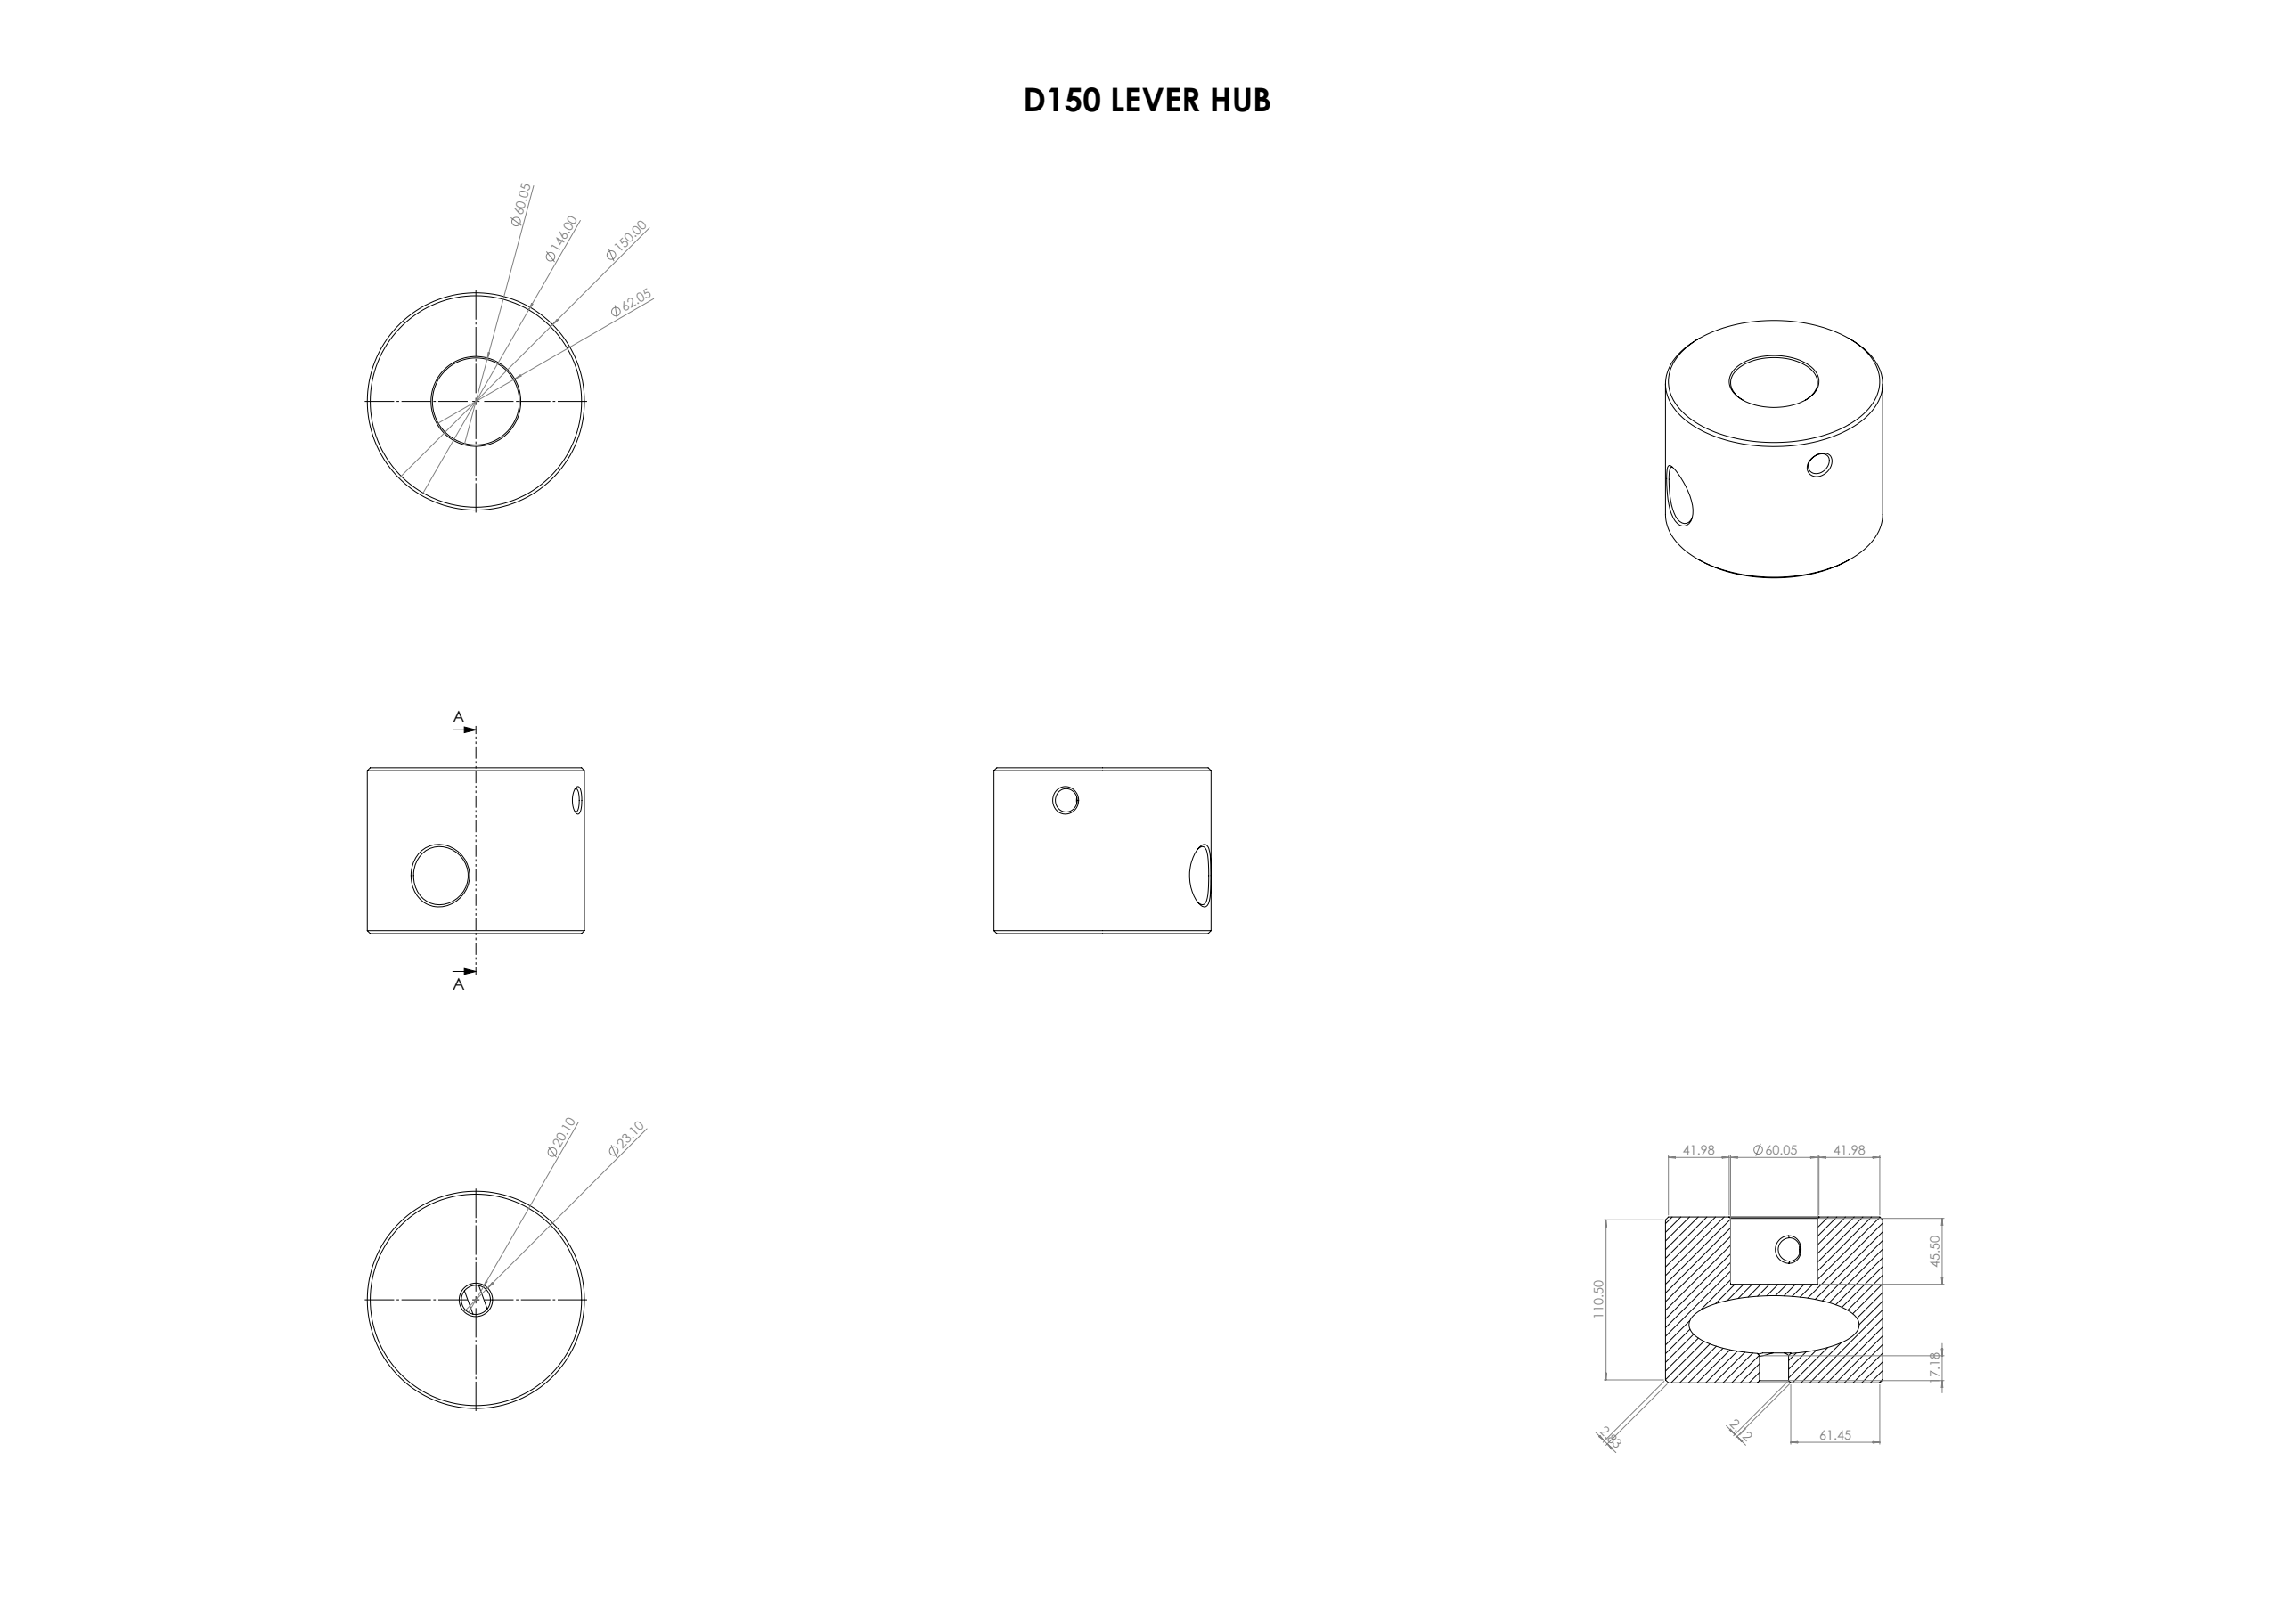
ISO-10303-21;
HEADER;
/* Generated by software containing ST-Developer
 * from STEP Tools, Inc. (www.steptools.com) 
 */

FILE_DESCRIPTION(
/* description */ (''),
/* implementation_level */ '2;1');

FILE_NAME(
/* name */ '04_D150_Lever_Hub.step',
/* time_stamp */ '2026-10-19T23:58:09-07:00',
/* author */ (''),
/* organization */ (''),
/* preprocessor_version */ 'ST-DEVELOPER v20.2',
/* originating_system */ 'Autodesk Translation Framework v15.15.0.0',
/* authorisation */ '');

FILE_SCHEMA (('AP203_CONFIGURATION_CONTROLLED_3D_DESIGN_OF_MECHANICAL_PARTS_AND_ASSEMBLIES_MIM_LF { 1 0 10303 203 3 1 4 }',
'AUTOMOTIVE_DESIGN { 1 0 10303 214 3 1 1 }','INTEGRATED_CNC_SCHEMA','MODEL_BASED_INTEGRATED_MANUFACTURING_SCHEMA',
'PROCESS_PLANNING_SCHEMA','AP242_MANAGED_MODEL_BASED_3D_ENGINEERING_MIM_LF { 1 0 10303 442 3 1 4 }'));
ENDSEC;

DATA;
#10=MECHANICAL_DESIGN_GEOMETRIC_PRESENTATION_REPRESENTATION('',(#417),#70757);
#280=B_SPLINE_SURFACE_WITH_KNOTS('',3,3,((#59484,#59485,#59486,#59487,#59488,
#59489,#59490,#59491,#59492,#59493,#59494,#59495,#59496,#59497,#59498,#59499,
#59500,#59501,#59502,#59503,#59504,#59505,#59506,#59507,#59508,#59509,#59510,
#59511,#59512,#59513,#59514,#59515,#59516,#59517,#59518,#59519,#59520,#59521,
#59522,#59523,#59524,#59525,#59526,#59527,#59528,#59529),(#59530,#59531,
#59532,#59533,#59534,#59535,#59536,#59537,#59538,#59539,#59540,#59541,#59542,
#59543,#59544,#59545,#59546,#59547,#59548,#59549,#59550,#59551,#59552,#59553,
#59554,#59555,#59556,#59557,#59558,#59559,#59560,#59561,#59562,#59563,#59564,
#59565,#59566,#59567,#59568,#59569,#59570,#59571,#59572,#59573,#59574,#59575),
(#59576,#59577,#59578,#59579,#59580,#59581,#59582,#59583,#59584,#59585,
#59586,#59587,#59588,#59589,#59590,#59591,#59592,#59593,#59594,#59595,#59596,
#59597,#59598,#59599,#59600,#59601,#59602,#59603,#59604,#59605,#59606,#59607,
#59608,#59609,#59610,#59611,#59612,#59613,#59614,#59615,#59616,#59617,#59618,
#59619,#59620,#59621),(#59622,#59623,#59624,#59625,#59626,#59627,#59628,
#59629,#59630,#59631,#59632,#59633,#59634,#59635,#59636,#59637,#59638,#59639,
#59640,#59641,#59642,#59643,#59644,#59645,#59646,#59647,#59648,#59649,#59650,
#59651,#59652,#59653,#59654,#59655,#59656,#59657,#59658,#59659,#59660,#59661,
#59662,#59663,#59664,#59665,#59666,#59667)),.UNSPECIFIED.,.F.,.T.,.F.,(4,
4),(4,1,1,1,1,1,1,1,1,1,1,1,1,1,1,1,1,1,1,1,1,1,1,1,1,1,1,1,1,1,1,1,1,1,
1,1,1,1,1,1,1,1,1,4),(0.,1.),(0.,0.434952646357303,0.869905292714605,1.08738161589326,
1.30485793907191,1.73981058542921,2.17476323178651,2.39223955496516,2.50097771655449,
2.55534679734915,2.60971587814382,3.04466852450112,3.15340668609044,3.47962117085842,
3.51586722472153,3.55211327858464,3.62460538631086,3.76958960176329,4.05955803266816,
4.34952646357303,4.6394948944779,4.92946332538276,5.21943175628763,5.5094001871925,
5.72687651037115,5.79936861809737,6.37930547990711,6.66927391081198,6.95924234171684,
7.24921077262171,7.53917920352658,7.82914763443145,8.11911606533632,8.26410028078875,
8.69905292714605,8.98902135805092,9.27898978895579,9.85892665076553,10.4388635125753,
10.8738161589326,10.9825543205219,11.3087688052899,11.7437214516472,12.1786740980045),
 .UNSPECIFIED.);
#281=B_SPLINE_SURFACE_WITH_KNOTS('',3,3,((#59965,#59966,#59967,#59968,#59969,
#59970,#59971,#59972,#59973,#59974,#59975,#59976,#59977,#59978,#59979,#59980,
#59981,#59982,#59983,#59984,#59985,#59986,#59987,#59988,#59989,#59990,#59991,
#59992,#59993,#59994,#59995,#59996,#59997,#59998,#59999,#60000,#60001,#60002,
#60003,#60004,#60005,#60006,#60007,#60008,#60009,#60010,#60011,#60012,#60013,
#60014,#60015,#60016,#60017,#60018),(#60019,#60020,#60021,#60022,#60023,
#60024,#60025,#60026,#60027,#60028,#60029,#60030,#60031,#60032,#60033,#60034,
#60035,#60036,#60037,#60038,#60039,#60040,#60041,#60042,#60043,#60044,#60045,
#60046,#60047,#60048,#60049,#60050,#60051,#60052,#60053,#60054,#60055,#60056,
#60057,#60058,#60059,#60060,#60061,#60062,#60063,#60064,#60065,#60066,#60067,
#60068,#60069,#60070,#60071,#60072),(#60073,#60074,#60075,#60076,#60077,
#60078,#60079,#60080,#60081,#60082,#60083,#60084,#60085,#60086,#60087,#60088,
#60089,#60090,#60091,#60092,#60093,#60094,#60095,#60096,#60097,#60098,#60099,
#60100,#60101,#60102,#60103,#60104,#60105,#60106,#60107,#60108,#60109,#60110,
#60111,#60112,#60113,#60114,#60115,#60116,#60117,#60118,#60119,#60120,#60121,
#60122,#60123,#60124,#60125,#60126),(#60127,#60128,#60129,#60130,#60131,
#60132,#60133,#60134,#60135,#60136,#60137,#60138,#60139,#60140,#60141,#60142,
#60143,#60144,#60145,#60146,#60147,#60148,#60149,#60150,#60151,#60152,#60153,
#60154,#60155,#60156,#60157,#60158,#60159,#60160,#60161,#60162,#60163,#60164,
#60165,#60166,#60167,#60168,#60169,#60170,#60171,#60172,#60173,#60174,#60175,
#60176,#60177,#60178,#60179,#60180)),.UNSPECIFIED.,.F.,.T.,.F.,(4,4),(4,
1,1,1,1,1,1,1,1,1,1,1,1,1,1,1,1,1,1,1,1,1,1,1,1,1,1,1,1,1,1,1,1,1,1,1,1,
1,1,1,1,1,1,1,1,1,1,1,1,1,1,4),(0.,1.),(0.,0.434952646357303,0.869905292714606,
1.08738161589326,1.30485793907191,1.73981058542921,1.84854874701854,2.17476323178651,
2.39223955496517,2.50097771655449,2.51456998675316,2.55534679734915,2.58253133774649,
2.60971587814382,2.88156128211713,3.04466852450112,3.47962117085842,3.51586722472153,
3.52492873818731,3.55211327858464,3.62460538631086,3.76958960176329,3.87832776335262,
4.05955803266816,4.34952646357303,4.6394948944779,4.85697121765655,4.92946332538276,
5.21943175628763,5.5094001871925,5.79936861809737,6.01684494127602,6.08933704900224,
6.37930547990711,6.95924234171684,7.03173444944306,7.24921077262171,7.53917920352658,
7.82914763443145,8.11911606533632,8.55406871169362,8.69905292714606,8.98902135805092,
9.27898978895579,9.64145032758688,9.85892665076553,10.4388635125753,10.8738161589326,
10.9825543205219,11.3087688052899,11.7437214516472,12.1786740980045),
 .UNSPECIFIED.);
#282=B_SPLINE_SURFACE_WITH_KNOTS('',3,3,((#60230,#60231,#60232,#60233,#60234,
#60235,#60236,#60237,#60238,#60239,#60240,#60241,#60242,#60243,#60244),
(#60245,#60246,#60247,#60248,#60249,#60250,#60251,#60252,#60253,#60254,
#60255,#60256,#60257,#60258,#60259),(#60260,#60261,#60262,#60263,#60264,
#60265,#60266,#60267,#60268,#60269,#60270,#60271,#60272,#60273,#60274),
(#60275,#60276,#60277,#60278,#60279,#60280,#60281,#60282,#60283,#60284,
#60285,#60286,#60287,#60288,#60289)),.UNSPECIFIED.,.F.,.F.,.F.,(4,4),(4,
1,1,1,1,1,1,1,2,2,4),(0.,1.),(0.442064469509103,0.769855887687593,1.09764730586608,
1.26154301495533,1.42543872404457,1.58933443313382,1.75323014222306,1.91712585131231,
2.08102156040155,2.14351932926336,2.6484237026181),.UNSPECIFIED.);
#283=B_SPLINE_SURFACE_WITH_KNOTS('',3,3,((#60302,#60303,#60304,#60305,#60306,
#60307,#60308,#60309,#60310,#60311,#60312,#60313,#60314,#60315),(#60316,
#60317,#60318,#60319,#60320,#60321,#60322,#60323,#60324,#60325,#60326,#60327,
#60328,#60329),(#60330,#60331,#60332,#60333,#60334,#60335,#60336,#60337,
#60338,#60339,#60340,#60341,#60342,#60343),(#60344,#60345,#60346,#60347,
#60348,#60349,#60350,#60351,#60352,#60353,#60354,#60355,#60356,#60357)),
 .UNSPECIFIED.,.F.,.F.,.F.,(4,4),(4,1,1,1,1,1,1,2,2,4),(0.,1.),(3.53272900796379,
3.8604875262342,4.18824604450462,4.35212530363983,4.51600456277503,4.72085363669404,
4.84376308104545,5.17152159931586,5.23401936817767,5.73877023945777),
 .UNSPECIFIED.);
#284=B_SPLINE_SURFACE_WITH_KNOTS('',3,3,((#60370,#60371,#60372,#60373,#60374,
#60375,#60376,#60377,#60378,#60379,#60380,#60381,#60382,#60383,#60384,#60385,
#60386,#60387,#60388,#60389,#60390,#60391,#60392,#60393),(#60394,#60395,
#60396,#60397,#60398,#60399,#60400,#60401,#60402,#60403,#60404,#60405,#60406,
#60407,#60408,#60409,#60410,#60411,#60412,#60413,#60414,#60415,#60416,#60417),
(#60418,#60419,#60420,#60421,#60422,#60423,#60424,#60425,#60426,#60427,
#60428,#60429,#60430,#60431,#60432,#60433,#60434,#60435,#60436,#60437,#60438,
#60439,#60440,#60441),(#60442,#60443,#60444,#60445,#60446,#60447,#60448,
#60449,#60450,#60451,#60452,#60453,#60454,#60455,#60456,#60457,#60458,#60459,
#60460,#60461,#60462,#60463,#60464,#60465)),.UNSPECIFIED.,.F.,.T.,.F.,(4,
4),(4,1,1,1,1,2,2,1,2,1,1,1,1,1,1,1,1,1,4),(0.,1.),(-3.74583112016425,-3.27642035446956,
-3.15906766304589,-2.80700958877487,-2.33759882308018,-1.86818805738549,
-1.79629199573878,-1.50783982646145,-1.21938765718412,-0.911365009587737,
-0.757353685789545,-0.603342361991352,-0.295319714394966,-0.141308390596773,
0.0127029332014201,0.320725580797806,0.628748228394192,0.936770875990578,
1.24479352358696),.UNSPECIFIED.);
#285=B_SPLINE_SURFACE_WITH_KNOTS('',3,3,((#60599,#60600,#60601,#60602,#60603,
#60604,#60605,#60606,#60607,#60608,#60609,#60610,#60611,#60612,#60613,#60614,
#60615,#60616,#60617,#60618,#60619,#60620,#60621,#60622,#60623,#60624,#60625,
#60626,#60627,#60628,#60629,#60630,#60631,#60632,#60633,#60634,#60635,#60636,
#60637,#60638,#60639,#60640,#60641,#60642,#60643,#60644,#60645,#60646,#60647,
#60648,#60649,#60650,#60651,#60652,#60653,#60654,#60655,#60656),(#60657,
#60658,#60659,#60660,#60661,#60662,#60663,#60664,#60665,#60666,#60667,#60668,
#60669,#60670,#60671,#60672,#60673,#60674,#60675,#60676,#60677,#60678,#60679,
#60680,#60681,#60682,#60683,#60684,#60685,#60686,#60687,#60688,#60689,#60690,
#60691,#60692,#60693,#60694,#60695,#60696,#60697,#60698,#60699,#60700,#60701,
#60702,#60703,#60704,#60705,#60706,#60707,#60708,#60709,#60710,#60711,#60712,
#60713,#60714),(#60715,#60716,#60717,#60718,#60719,#60720,#60721,#60722,
#60723,#60724,#60725,#60726,#60727,#60728,#60729,#60730,#60731,#60732,#60733,
#60734,#60735,#60736,#60737,#60738,#60739,#60740,#60741,#60742,#60743,#60744,
#60745,#60746,#60747,#60748,#60749,#60750,#60751,#60752,#60753,#60754,#60755,
#60756,#60757,#60758,#60759,#60760,#60761,#60762,#60763,#60764,#60765,#60766,
#60767,#60768,#60769,#60770,#60771,#60772),(#60773,#60774,#60775,#60776,
#60777,#60778,#60779,#60780,#60781,#60782,#60783,#60784,#60785,#60786,#60787,
#60788,#60789,#60790,#60791,#60792,#60793,#60794,#60795,#60796,#60797,#60798,
#60799,#60800,#60801,#60802,#60803,#60804,#60805,#60806,#60807,#60808,#60809,
#60810,#60811,#60812,#60813,#60814,#60815,#60816,#60817,#60818,#60819,#60820,
#60821,#60822,#60823,#60824,#60825,#60826,#60827,#60828,#60829,#60830)),
 .UNSPECIFIED.,.F.,.T.,.F.,(4,4),(4,1,1,1,1,1,1,1,1,1,1,1,1,1,1,1,1,1,1,
1,1,1,1,1,1,1,1,1,1,1,1,1,1,1,1,1,1,1,1,1,1,1,1,1,1,1,1,1,1,1,1,1,1,1,1,
4),(0.,1.),(0.,0.173419326361772,0.346838652723544,0.520257979085315,0.693677305447087,
0.867096631808859,0.953806294989745,0.997161126580188,1.04051595817063,
1.38735461089417,1.41625783195447,1.44516105301476,1.50296749513536,1.61858037937654,
1.73419326361772,1.8498061478589,2.08103191634126,2.10993513740156,2.13883835846185,
2.19664480058244,2.25445124270303,2.28335446376333,2.31225768482362,2.54348345330599,
2.57238667436628,2.60128989542658,2.65909633754717,2.77470922178835,2.94812854815012,
3.12154787451189,3.20825753769278,3.29496720087366,3.38167686405455,3.39251557195216,
3.40335427984977,3.42503169564499,3.4358704035426,3.44670911144021,3.45754781933783,
3.46296717328663,3.46838652723544,3.64180585359721,3.81522517995898,3.82606388785659,
3.8369025957542,3.85858001154942,3.90193484313987,3.98864450632075,4.07535416950164,
4.16206383268252,4.33548315904429,4.35716057483952,4.37883799063474,4.42219282222518,
4.50890248540607,4.85574113812961),.UNSPECIFIED.);
#387=SHAPE_REPRESENTATION_RELATIONSHIP('SRR','None',#70828,#402);
#402=ADVANCED_BREP_SHAPE_REPRESENTATION('',(#477),#70752);
#417=STYLED_ITEM('',(#71033),#477);
#477=MANIFOLD_SOLID_BREP('Hub',#26882);
#723=CYLINDRICAL_SURFACE('',#27792,7.5);
#724=CYLINDRICAL_SURFACE('',#27795,2.01);
#725=CYLINDRICAL_SURFACE('',#27799,1.005);
#726=CYLINDRICAL_SURFACE('',#27805,0.805000000000009);
#727=CYLINDRICAL_SURFACE('',#27806,3.0025);
#868=FACE_BOUND('',#4617,.T.);
#869=FACE_BOUND('',#4618,.T.);
#870=FACE_BOUND('',#4619,.T.);
#871=FACE_BOUND('',#4621,.T.);
#872=FACE_BOUND('',#4626,.T.);
#873=FACE_BOUND('',#4632,.T.);
#874=FACE_BOUND('',#4639,.T.);
#1376=B_SPLINE_CURVE_WITH_KNOTS('',3,(#59671,#59672,#59673,#59674,#59675,
#59676,#59677,#59678,#59679,#59680,#59681,#59682,#59683,#59684,#59685,#59686,
#59687,#59688,#59689,#59690,#59691,#59692,#59693,#59694,#59695,#59696,#59697,
#59698,#59699,#59700,#59701,#59702,#59703,#59704,#59705,#59706,#59707,#59708,
#59709,#59710,#59711,#59712,#59713,#59714,#59715,#59716),.UNSPECIFIED.,
 .T.,.F.,(4,1,1,1,1,1,1,1,1,1,1,1,1,1,1,1,1,1,1,1,1,1,1,1,1,1,1,1,1,1,1,
1,1,1,1,1,1,1,1,1,1,1,1,4),(0.,0.434952646357303,0.869905292714605,1.08738161589326,
1.30485793907191,1.73981058542921,2.17476323178651,2.39223955496516,2.50097771655449,
2.55534679734915,2.60971587814382,3.04466852450112,3.15340668609044,3.47962117085842,
3.51586722472153,3.55211327858464,3.62460538631086,3.76958960176329,4.05955803266816,
4.34952646357303,4.6394948944779,4.92946332538276,5.21943175628763,5.5094001871925,
5.72687651037115,5.79936861809737,6.37930547990711,6.66927391081198,6.95924234171684,
7.24921077262171,7.53917920352658,7.82914763443145,8.11911606533632,8.26410028078875,
8.69905292714605,8.98902135805092,9.27898978895579,9.85892665076553,10.4388635125753,
10.8738161589326,10.9825543205219,11.3087688052899,11.7437214516472,12.1786740980045),
 .UNSPECIFIED.);
#1377=B_SPLINE_CURVE_WITH_KNOTS('',3,(#59717,#59718,#59719,#59720,#59721,
#59722,#59723,#59724,#59725,#59726,#59727,#59728,#59729,#59730,#59731,#59732,
#59733,#59734,#59735,#59736,#59737,#59738,#59739,#59740,#59741,#59742,#59743,
#59744,#59745,#59746,#59747,#59748,#59749,#59750,#59751,#59752,#59753,#59754,
#59755,#59756,#59757,#59758,#59759,#59760,#59761,#59762),.UNSPECIFIED.,
 .T.,.F.,(4,1,1,1,1,1,1,1,1,1,1,1,1,1,1,1,1,1,1,1,1,1,1,1,1,1,1,1,1,1,1,
1,1,1,1,1,1,1,1,1,1,1,1,4),(-12.1786740980045,-11.7437214516472,-11.3087688052899,
-10.9825543205219,-10.8738161589326,-10.4388635125753,-9.85892665076553,
-9.27898978895579,-8.98902135805092,-8.69905292714605,-8.26410028078875,
-8.11911606533632,-7.82914763443145,-7.53917920352658,-7.24921077262171,
-6.95924234171684,-6.66927391081198,-6.37930547990711,-5.79936861809737,
-5.72687651037115,-5.5094001871925,-5.21943175628763,-4.92946332538276,
-4.6394948944779,-4.34952646357303,-4.05955803266816,-3.76958960176329,
-3.62460538631086,-3.55211327858464,-3.51586722472153,-3.47962117085842,
-3.15340668609044,-3.04466852450112,-2.60971587814382,-2.55534679734915,
-2.50097771655449,-2.39223955496516,-2.17476323178651,-1.73981058542921,
-1.30485793907191,-1.08738161589326,-0.869905292714605,-0.434952646357303,
0.),.UNSPECIFIED.);
#1378=B_SPLINE_CURVE_WITH_KNOTS('',3,(#59770,#59771,#59772,#59773,#59774,
#59775,#59776,#59777,#59778,#59779,#59780,#59781,#59782,#59783,#59784,#59785,
#59786,#59787,#59788,#59789,#59790,#59791,#59792,#59793,#59794,#59795,#59796,
#59797,#59798,#59799,#59800,#59801,#59802,#59803,#59804,#59805,#59806,#59807,
#59808,#59809,#59810,#59811,#59812,#59813,#59814,#59815,#59816,#59817,#59818,
#59819,#59820,#59821,#59822,#59823),.UNSPECIFIED.,.T.,.F.,(4,1,1,1,1,1,
1,1,1,1,1,1,1,1,1,1,1,1,1,1,1,1,1,1,1,1,1,1,1,1,1,1,1,1,1,1,1,1,1,1,1,1,
1,1,1,1,1,1,1,1,1,4),(-12.1786740980045,-11.7437214516472,-11.3087688052899,
-10.9825543205219,-10.8738161589326,-10.4388635125753,-9.85892665076553,
-9.64145032758688,-9.27898978895579,-8.98902135805092,-8.69905292714606,
-8.55406871169362,-8.11911606533632,-7.82914763443145,-7.53917920352658,
-7.24921077262171,-7.03173444944306,-6.95924234171684,-6.37930547990711,
-6.08933704900224,-6.01684494127602,-5.79936861809737,-5.5094001871925,
-5.21943175628763,-4.92946332538276,-4.85697121765655,-4.6394948944779,
-4.34952646357303,-4.05955803266816,-3.87832776335262,-3.76958960176329,
-3.62460538631086,-3.55211327858464,-3.52492873818731,-3.51586722472153,
-3.47962117085842,-3.04466852450112,-2.88156128211713,-2.60971587814382,
-2.58253133774649,-2.55534679734915,-2.51456998675316,-2.50097771655449,
-2.39223955496517,-2.17476323178651,-1.84854874701854,-1.73981058542921,
-1.30485793907191,-1.08738161589326,-0.869905292714606,-0.434952646357303,
0.),.UNSPECIFIED.);
#1379=B_SPLINE_CURVE_WITH_KNOTS('',3,(#59825,#59826,#59827,#59828,#59829,
#59830,#59831,#59832,#59833,#59834,#59835,#59836,#59837,#59838,#59839,#59840,
#59841,#59842,#59843,#59844,#59845,#59846,#59847,#59848,#59849,#59850,#59851,
#59852,#59853,#59854,#59855,#59856,#59857,#59858,#59859,#59860,#59861,#59862,
#59863,#59864,#59865,#59866,#59867,#59868,#59869,#59870,#59871,#59872,#59873,
#59874,#59875,#59876,#59877,#59878,#59879,#59880,#59881,#59882),
 .UNSPECIFIED.,.T.,.F.,(4,1,1,1,1,1,1,1,1,1,1,1,1,1,1,1,1,1,1,1,1,1,1,1,
1,1,1,1,1,1,1,1,1,1,1,1,1,1,1,1,1,1,1,1,1,1,1,1,1,1,1,1,1,1,1,4),(-4.85574113812961,
-4.50890248540607,-4.42219282222518,-4.37883799063474,-4.35716057483952,
-4.33548315904429,-4.16206383268252,-4.07535416950164,-3.98864450632075,
-3.90193484313987,-3.85858001154942,-3.8369025957542,-3.82606388785659,
-3.81522517995898,-3.64180585359721,-3.46838652723544,-3.46296717328663,
-3.45754781933783,-3.44670911144021,-3.4358704035426,-3.42503169564499,
-3.40335427984977,-3.39251557195216,-3.38167686405455,-3.29496720087366,
-3.20825753769278,-3.12154787451189,-2.94812854815012,-2.77470922178835,
-2.65909633754717,-2.60128989542658,-2.57238667436628,-2.54348345330599,
-2.31225768482362,-2.28335446376333,-2.25445124270303,-2.19664480058244,
-2.13883835846185,-2.10993513740156,-2.08103191634126,-1.8498061478589,
-1.73419326361772,-1.61858037937654,-1.50296749513536,-1.44516105301476,
-1.41625783195447,-1.38735461089417,-1.04051595817063,-0.997161126580188,
-0.953806294989745,-0.867096631808859,-0.693677305447087,-0.520257979085315,
-0.346838652723544,-0.173419326361772,0.),.UNSPECIFIED.);
#1380=B_SPLINE_CURVE_WITH_KNOTS('',3,(#59886,#59887,#59888,#59889,#59890,
#59891,#59892,#59893,#59894,#59895,#59896,#59897,#59898,#59899,#59900,#59901,
#59902,#59903,#59904,#59905,#59906,#59907,#59908,#59909,#59910,#59911,#59912,
#59913,#59914,#59915,#59916,#59917,#59918,#59919,#59920,#59921,#59922,#59923,
#59924,#59925,#59926,#59927,#59928,#59929,#59930,#59931,#59932,#59933,#59934,
#59935,#59936,#59937,#59938,#59939),.UNSPECIFIED.,.T.,.F.,(4,1,1,1,1,1,
1,1,1,1,1,1,1,1,1,1,1,1,1,1,1,1,1,1,1,1,1,1,1,1,1,1,1,1,1,1,1,1,1,1,1,1,
1,1,1,1,1,1,1,1,1,4),(0.,0.434952646357303,0.869905292714606,1.08738161589326,
1.30485793907191,1.73981058542921,1.84854874701854,2.17476323178651,2.39223955496517,
2.50097771655449,2.51456998675316,2.55534679734915,2.58253133774649,2.60971587814382,
2.88156128211713,3.04466852450112,3.47962117085842,3.51586722472153,3.52492873818731,
3.55211327858464,3.62460538631086,3.76958960176329,3.87832776335262,4.05955803266816,
4.34952646357303,4.6394948944779,4.85697121765655,4.92946332538276,5.21943175628763,
5.5094001871925,5.79936861809737,6.01684494127602,6.08933704900224,6.37930547990711,
6.95924234171684,7.03173444944306,7.24921077262171,7.53917920352658,7.82914763443145,
8.11911606533632,8.55406871169362,8.69905292714606,8.98902135805092,9.27898978895579,
9.64145032758688,9.85892665076553,10.4388635125753,10.8738161589326,10.9825543205219,
11.3087688052899,11.7437214516472,12.1786740980045),.UNSPECIFIED.);
#1381=B_SPLINE_CURVE_WITH_KNOTS('',3,(#59944,#59945,#59946,#59947,#59948,
#59949,#59950,#59951,#59952),.UNSPECIFIED.,.F.,.F.,(4,1,1,1,1,1,4),(-5.09886318526994,
-4.84376308104545,-4.72085363669404,-4.51600456277503,-4.35212530363983,
-4.18824604450462,-4.17262768684822),.UNSPECIFIED.);
#1382=B_SPLINE_CURVE_WITH_KNOTS('',3,(#59955,#59956,#59957,#59958,#59959,
#59960,#59961,#59962,#59963,#59964),.UNSPECIFIED.,.F.,.F.,(4,1,1,1,1,1,
1,4),(-2.00844283647624,-1.91712585131231,-1.75323014222306,-1.58933443313382,
-1.42543872404457,-1.26154301495533,-1.09764730586608,-1.08195609140638),
 .UNSPECIFIED.);
#1383=B_SPLINE_CURVE_WITH_KNOTS('',3,(#60191,#60192,#60193,#60194,#60195,
#60196,#60197,#60198,#60199,#60200,#60201,#60202,#60203,#60204,#60205),
 .UNSPECIFIED.,.F.,.F.,(4,1,1,1,1,1,1,1,2,2,4),(0.442064469509103,0.769855887687593,
1.09764730586608,1.26154301495533,1.42543872404457,1.58933443313382,1.75323014222306,
1.91712585131231,2.08102156040155,2.14351932926336,2.6484237026181),
 .UNSPECIFIED.);
#1384=B_SPLINE_CURVE_WITH_KNOTS('',3,(#60209,#60210,#60211,#60212,#60213,
#60214,#60215,#60216,#60217,#60218,#60219,#60220,#60221,#60222),
 .UNSPECIFIED.,.F.,.F.,(4,1,1,1,1,1,1,2,2,4),(3.53272900796379,3.8604875262342,
4.18824604450462,4.35212530363983,4.51600456277503,4.72085363669404,4.84376308104545,
5.17152159931586,5.23401936817767,5.73877023945777),.UNSPECIFIED.);
#1385=B_SPLINE_CURVE_WITH_KNOTS('',3,(#60290,#60291,#60292,#60293,#60294,
#60295),.UNSPECIFIED.,.F.,.F.,(4,2,4),(0.,0.395295738561713,0.750556975338415),
 .UNSPECIFIED.);
#1386=B_SPLINE_CURVE_WITH_KNOTS('',3,(#60296,#60297,#60298,#60299,#60300,
#60301),.UNSPECIFIED.,.F.,.F.,(4,2,4),(0.,0.242165599626981,0.747632926534989),
 .UNSPECIFIED.);
#1387=B_SPLINE_CURVE_WITH_KNOTS('',3,(#60358,#60359,#60360,#60361,#60362,
#60363),.UNSPECIFIED.,.F.,.F.,(4,2,4),(0.,0.395285417853985,0.750556986687262),
 .UNSPECIFIED.);
#1388=B_SPLINE_CURVE_WITH_KNOTS('',3,(#60364,#60365,#60366,#60367,#60368,
#60369),.UNSPECIFIED.,.F.,.F.,(4,2,4),(0.,0.242119658779455,0.747632520146835),
 .UNSPECIFIED.);
#1389=B_SPLINE_CURVE_WITH_KNOTS('',3,(#60470,#60471,#60472,#60473,#60474,
#60475,#60476,#60477,#60478,#60479,#60480,#60481,#60482,#60483,#60484,#60485,
#60486,#60487,#60488,#60489,#60490),.UNSPECIFIED.,.F.,.F.,(4,1,1,1,1,2,
2,1,2,1,1,1,1,1,1,4),(-3.74583112016425,-3.27642035446956,-3.15906766304589,
-2.80700958877487,-2.33759882308018,-1.86818805738549,-1.79629199573878,
-1.50783982646145,-1.21938765718412,-0.911365009587737,-0.757353685789545,
-0.603342361991352,-0.295319714394966,-0.141308390596773,0.0127029332014201,
0.0186613584180625),.UNSPECIFIED.);
#1390=B_SPLINE_CURVE_WITH_KNOTS('',3,(#60491,#60492,#60493,#60494,#60495,
#60496,#60497),.UNSPECIFIED.,.F.,.F.,(4,1,1,1,4),(0.0186613584180625,0.320725580797806,
0.628748228394192,0.936770875990578,1.24479352358696),.UNSPECIFIED.);
#1391=B_SPLINE_CURVE_WITH_KNOTS('',3,(#60499,#60500,#60501,#60502,#60503,
#60504,#60505,#60506,#60507,#60508,#60509),.UNSPECIFIED.,.F.,.F.,(4,1,1,
1,1,1,1,1,4),(-1.24479352358696,-0.936770875990578,-0.628748228394192,-0.320725580797806,
-0.0127029332014201,0.141308390596773,0.295319714394966,0.603342361991352,
0.74818116877789),.UNSPECIFIED.);
#1392=B_SPLINE_CURVE_WITH_KNOTS('',3,(#60511,#60512,#60513,#60514,#60515,
#60516,#60517,#60518,#60519),.UNSPECIFIED.,.F.,.F.,(4,1,1,2,1,4),(0.74818116877789,
0.757353685789545,0.911365009587737,1.21938765718412,1.50783982646145,1.69059414559038),
 .UNSPECIFIED.);
#1393=B_SPLINE_CURVE_WITH_KNOTS('',3,(#60520,#60521,#60522,#60523,#60524,
#60525,#60526,#60527,#60528,#60529,#60530,#60531),.UNSPECIFIED.,.F.,.F.,
(4,2,2,1,1,1,1,4),(1.69059414559038,1.79629199573878,1.86818805738549,2.33759882308018,
2.80700958877487,3.15906766304589,3.27642035446956,3.74583112016425),
 .UNSPECIFIED.);
#1394=B_SPLINE_CURVE_WITH_KNOTS('',3,(#60534,#60535,#60536,#60537,#60538,
#60539,#60540,#60541,#60542,#60543,#60544,#60545,#60546,#60547,#60548,#60549,
#60550,#60551,#60552,#60553,#60554,#60555,#60556,#60557,#60558,#60559,#60560,
#60561,#60562,#60563,#60564,#60565,#60566,#60567,#60568,#60569,#60570,#60571,
#60572,#60573,#60574,#60575,#60576,#60577,#60578,#60579,#60580,#60581,#60582,
#60583,#60584,#60585,#60586,#60587,#60588,#60589,#60590,#60591),
 .UNSPECIFIED.,.T.,.F.,(4,1,1,1,1,1,1,1,1,1,1,1,1,1,1,1,1,1,1,1,1,1,1,1,
1,1,1,1,1,1,1,1,1,1,1,1,1,1,1,1,1,1,1,1,1,1,1,1,1,1,1,1,1,1,1,4),(0.,0.173419326361772,
0.346838652723544,0.520257979085315,0.693677305447087,0.867096631808859,
0.953806294989745,0.997161126580188,1.04051595817063,1.38735461089417,1.41625783195447,
1.44516105301476,1.50296749513536,1.61858037937654,1.73419326361772,1.8498061478589,
2.08103191634126,2.10993513740156,2.13883835846185,2.19664480058244,2.25445124270303,
2.28335446376333,2.31225768482362,2.54348345330599,2.57238667436628,2.60128989542658,
2.65909633754717,2.77470922178835,2.94812854815012,3.12154787451189,3.20825753769278,
3.29496720087366,3.38167686405455,3.39251557195216,3.40335427984977,3.42503169564499,
3.4358704035426,3.44670911144021,3.45754781933783,3.46296717328663,3.46838652723544,
3.64180585359721,3.81522517995898,3.82606388785659,3.8369025957542,3.85858001154942,
3.90193484313987,3.98864450632075,4.07535416950164,4.16206383268252,4.33548315904429,
4.35716057483952,4.37883799063474,4.42219282222518,4.50890248540607,4.85574113812961),
 .UNSPECIFIED.);
#1911=PLANE('',#27803);
#1912=PLANE('',#27809);
#1913=PLANE('',#27810);
#1914=PLANE('',#27811);
#1915=PLANE('',#27814);
#3103=FACE_OUTER_BOUND('',#4615,.T.);
#3104=FACE_OUTER_BOUND('',#4616,.T.);
#3105=FACE_OUTER_BOUND('',#4620,.T.);
#3106=FACE_OUTER_BOUND('',#4622,.T.);
#3107=FACE_OUTER_BOUND('',#4623,.T.);
#3108=FACE_OUTER_BOUND('',#4624,.T.);
#3109=FACE_OUTER_BOUND('',#4625,.T.);
#3110=FACE_OUTER_BOUND('',#4627,.T.);
#3111=FACE_OUTER_BOUND('',#4628,.T.);
#3112=FACE_OUTER_BOUND('',#4629,.T.);
#3113=FACE_OUTER_BOUND('',#4630,.T.);
#3114=FACE_OUTER_BOUND('',#4631,.T.);
#3115=FACE_OUTER_BOUND('',#4633,.T.);
#3116=FACE_OUTER_BOUND('',#4634,.T.);
#3117=FACE_OUTER_BOUND('',#4635,.T.);
#3118=FACE_OUTER_BOUND('',#4636,.T.);
#3119=FACE_OUTER_BOUND('',#4637,.T.);
#3120=FACE_OUTER_BOUND('',#4638,.T.);
#3121=FACE_OUTER_BOUND('',#4640,.T.);
#3122=FACE_OUTER_BOUND('',#4641,.T.);
#4615=EDGE_LOOP('',(#20248,#20249,#20250,#20251));
#4616=EDGE_LOOP('',(#20252,#20253,#20254,#20255));
#4617=EDGE_LOOP('',(#20256));
#4618=EDGE_LOOP('',(#20257));
#4619=EDGE_LOOP('',(#20258));
#4620=EDGE_LOOP('',(#20259,#20260,#20261,#20262));
#4621=EDGE_LOOP('',(#20263,#20264,#20265,#20266));
#4622=EDGE_LOOP('',(#20267,#20268,#20269,#20270));
#4623=EDGE_LOOP('',(#20271,#20272,#20273,#20274));
#4624=EDGE_LOOP('',(#20275,#20276,#20277,#20278,#20279,#20280,#20281,#20282));
#4625=EDGE_LOOP('',(#20283));
#4626=EDGE_LOOP('',(#20284));
#4627=EDGE_LOOP('',(#20285,#20286,#20287,#20288));
#4628=EDGE_LOOP('',(#20289,#20290,#20291,#20292));
#4629=EDGE_LOOP('',(#20293,#20294,#20295,#20296,#20297,#20298,#20299));
#4630=EDGE_LOOP('',(#20300,#20301,#20302,#20303,#20304));
#4631=EDGE_LOOP('',(#20305,#20306,#20307,#20308));
#4632=EDGE_LOOP('',(#20309,#20310,#20311));
#4633=EDGE_LOOP('',(#20312,#20313,#20314,#20315));
#4634=EDGE_LOOP('',(#20316,#20317,#20318,#20319,#20320));
#4635=EDGE_LOOP('',(#20321,#20322,#20323,#20324));
#4636=EDGE_LOOP('',(#20325));
#4637=EDGE_LOOP('',(#20326,#20327,#20328,#20329));
#4638=EDGE_LOOP('',(#20330));
#4639=EDGE_LOOP('',(#20331));
#4640=EDGE_LOOP('',(#20332,#20333,#20334,#20335));
#4641=EDGE_LOOP('',(#20336,#20337,#20338,#20339));
#6234=LINE('',#59670,#8731);
#6235=LINE('',#59767,#8732);
#6236=LINE('',#59885,#8733);
#6237=LINE('',#59942,#8734);
#6238=LINE('',#59954,#8735);
#6239=LINE('',#60181,#8736);
#6240=LINE('',#60186,#8737);
#6241=LINE('',#60225,#8738);
#6242=LINE('',#60468,#8739);
#6243=LINE('',#60592,#8740);
#6244=LINE('',#60597,#8741);
#6245=LINE('',#60831,#8742);
#6246=LINE('',#60837,#8743);
#6247=LINE('',#60843,#8744);
#6248=LINE('',#60845,#8745);
#8731=VECTOR('',#31067,1.);
#8732=VECTOR('',#31072,7.5);
#8733=VECTOR('',#31077,2.01);
#8734=VECTOR('',#31078,1.);
#8735=VECTOR('',#31079,1.);
#8736=VECTOR('',#31080,1.);
#8737=VECTOR('',#31085,1.08);
#8738=VECTOR('',#31094,1.005);
#8739=VECTOR('',#31101,1.);
#8740=VECTOR('',#31104,0.805000000000009);
#8741=VECTOR('',#31109,3.0025);
#8742=VECTOR('',#31112,1.);
#8743=VECTOR('',#31121,3.0525);
#8744=VECTOR('',#31130,7.4);
#8745=VECTOR('',#31133,7.4);
#10864=CIRCLE('',#27793,7.5);
#10865=CIRCLE('',#27794,7.5);
#10866=CIRCLE('',#27797,1.155);
#10867=CIRCLE('',#27798,1.005);
#10868=CIRCLE('',#27800,1.005);
#10869=CIRCLE('',#27801,1.005);
#10870=CIRCLE('',#27802,1.005);
#10871=CIRCLE('',#27804,7.3);
#10872=CIRCLE('',#27807,3.0025);
#10873=CIRCLE('',#27808,3.0025);
#10874=CIRCLE('',#27813,3.1025);
#10875=CIRCLE('',#27815,7.3);
#12004=VERTEX_POINT('',#59668);
#12005=VERTEX_POINT('',#59669);
#12006=VERTEX_POINT('',#59764);
#12007=VERTEX_POINT('',#59766);
#12008=VERTEX_POINT('',#59769);
#12009=VERTEX_POINT('',#59824);
#12010=VERTEX_POINT('',#59884);
#12011=VERTEX_POINT('',#59940);
#12012=VERTEX_POINT('',#59941);
#12013=VERTEX_POINT('',#59943);
#12014=VERTEX_POINT('',#59953);
#12015=VERTEX_POINT('',#60183);
#12016=VERTEX_POINT('',#60185);
#12017=VERTEX_POINT('',#60189);
#12018=VERTEX_POINT('',#60190);
#12019=VERTEX_POINT('',#60206);
#12020=VERTEX_POINT('',#60208);
#12021=VERTEX_POINT('',#60223);
#12022=VERTEX_POINT('',#60228);
#12023=VERTEX_POINT('',#60466);
#12024=VERTEX_POINT('',#60467);
#12025=VERTEX_POINT('',#60469);
#12026=VERTEX_POINT('',#60498);
#12027=VERTEX_POINT('',#60510);
#12028=VERTEX_POINT('',#60533);
#12029=VERTEX_POINT('',#60594);
#12030=VERTEX_POINT('',#60596);
#12031=VERTEX_POINT('',#60836);
#12032=VERTEX_POINT('',#60840);
#14977=EDGE_CURVE('',#12004,#12005,#6234,.T.);
#14978=EDGE_CURVE('',#12005,#12005,#1376,.T.);
#14979=EDGE_CURVE('',#12004,#12004,#1377,.T.);
#14980=EDGE_CURVE('',#12006,#12006,#10864,.T.);
#14981=EDGE_CURVE('',#12006,#12007,#6235,.T.);
#14982=EDGE_CURVE('',#12007,#12007,#10865,.T.);
#14983=EDGE_CURVE('',#12008,#12008,#1378,.T.);
#14984=EDGE_CURVE('',#12009,#12009,#1379,.T.);
#14985=EDGE_CURVE('',#12005,#12010,#6236,.T.);
#14986=EDGE_CURVE('',#12010,#12010,#1380,.T.);
#14987=EDGE_CURVE('',#12011,#12012,#6237,.T.);
#14988=EDGE_CURVE('',#12013,#12012,#1381,.T.);
#14989=EDGE_CURVE('',#12013,#12014,#6238,.T.);
#14990=EDGE_CURVE('',#12011,#12014,#1382,.T.);
#14991=EDGE_CURVE('',#12008,#12010,#6239,.T.);
#14992=EDGE_CURVE('',#12015,#12015,#10866,.T.);
#14993=EDGE_CURVE('',#12015,#12016,#6240,.T.);
#14994=EDGE_CURVE('',#12016,#12016,#10867,.T.);
#14995=EDGE_CURVE('',#12017,#12018,#1383,.T.);
#14996=EDGE_CURVE('',#12019,#12017,#10868,.T.);
#14997=EDGE_CURVE('',#12020,#12019,#1384,.T.);
#14998=EDGE_CURVE('',#12021,#12020,#10869,.T.);
#14999=EDGE_CURVE('',#12021,#12016,#6241,.T.);
#15000=EDGE_CURVE('',#12018,#12021,#10870,.T.);
#15001=EDGE_CURVE('',#12022,#12022,#10871,.T.);
#15002=EDGE_CURVE('',#12014,#12017,#1385,.F.);
#15003=EDGE_CURVE('',#12018,#12011,#1386,.F.);
#15004=EDGE_CURVE('',#12012,#12020,#1387,.F.);
#15005=EDGE_CURVE('',#12019,#12013,#1388,.F.);
#15006=EDGE_CURVE('',#12023,#12024,#6242,.T.);
#15007=EDGE_CURVE('',#12024,#12025,#1389,.T.);
#15008=EDGE_CURVE('',#12025,#12024,#1390,.T.);
#15009=EDGE_CURVE('',#12023,#12026,#1391,.T.);
#15010=EDGE_CURVE('',#12026,#12027,#1392,.T.);
#15011=EDGE_CURVE('',#12027,#12023,#1393,.T.);
#15012=EDGE_CURVE('',#12028,#12028,#1394,.T.);
#15013=EDGE_CURVE('',#12028,#12025,#6243,.T.);
#15014=EDGE_CURVE('',#12029,#12029,#10872,.T.);
#15015=EDGE_CURVE('',#12029,#12030,#6244,.T.);
#15016=EDGE_CURVE('',#12030,#12030,#10873,.T.);
#15017=EDGE_CURVE('',#12009,#12028,#6245,.T.);
#15018=EDGE_CURVE('',#12030,#12031,#6246,.T.);
#15019=EDGE_CURVE('',#12031,#12031,#10874,.T.);
#15020=EDGE_CURVE('',#12032,#12032,#10875,.T.);
#15021=EDGE_CURVE('',#12007,#12032,#6247,.T.);
#15022=EDGE_CURVE('',#12022,#12006,#6248,.T.);
#20248=ORIENTED_EDGE('',*,*,#14977,.T.);
#20249=ORIENTED_EDGE('',*,*,#14978,.T.);
#20250=ORIENTED_EDGE('',*,*,#14977,.F.);
#20251=ORIENTED_EDGE('',*,*,#14979,.T.);
#20252=ORIENTED_EDGE('',*,*,#14980,.F.);
#20253=ORIENTED_EDGE('',*,*,#14981,.T.);
#20254=ORIENTED_EDGE('',*,*,#14982,.T.);
#20255=ORIENTED_EDGE('',*,*,#14981,.F.);
#20256=ORIENTED_EDGE('',*,*,#14983,.F.);
#20257=ORIENTED_EDGE('',*,*,#14984,.F.);
#20258=ORIENTED_EDGE('',*,*,#14979,.F.);
#20259=ORIENTED_EDGE('',*,*,#14978,.F.);
#20260=ORIENTED_EDGE('',*,*,#14985,.T.);
#20261=ORIENTED_EDGE('',*,*,#14986,.F.);
#20262=ORIENTED_EDGE('',*,*,#14985,.F.);
#20263=ORIENTED_EDGE('',*,*,#14987,.T.);
#20264=ORIENTED_EDGE('',*,*,#14988,.F.);
#20265=ORIENTED_EDGE('',*,*,#14989,.T.);
#20266=ORIENTED_EDGE('',*,*,#14990,.F.);
#20267=ORIENTED_EDGE('',*,*,#14991,.T.);
#20268=ORIENTED_EDGE('',*,*,#14986,.T.);
#20269=ORIENTED_EDGE('',*,*,#14991,.F.);
#20270=ORIENTED_EDGE('',*,*,#14983,.T.);
#20271=ORIENTED_EDGE('',*,*,#14992,.T.);
#20272=ORIENTED_EDGE('',*,*,#14993,.T.);
#20273=ORIENTED_EDGE('',*,*,#14994,.T.);
#20274=ORIENTED_EDGE('',*,*,#14993,.F.);
#20275=ORIENTED_EDGE('',*,*,#14995,.F.);
#20276=ORIENTED_EDGE('',*,*,#14996,.F.);
#20277=ORIENTED_EDGE('',*,*,#14997,.F.);
#20278=ORIENTED_EDGE('',*,*,#14998,.F.);
#20279=ORIENTED_EDGE('',*,*,#14999,.T.);
#20280=ORIENTED_EDGE('',*,*,#14994,.F.);
#20281=ORIENTED_EDGE('',*,*,#14999,.F.);
#20282=ORIENTED_EDGE('',*,*,#15000,.F.);
#20283=ORIENTED_EDGE('',*,*,#15001,.T.);
#20284=ORIENTED_EDGE('',*,*,#14992,.F.);
#20285=ORIENTED_EDGE('',*,*,#15002,.T.);
#20286=ORIENTED_EDGE('',*,*,#14995,.T.);
#20287=ORIENTED_EDGE('',*,*,#15003,.T.);
#20288=ORIENTED_EDGE('',*,*,#14990,.T.);
#20289=ORIENTED_EDGE('',*,*,#15004,.T.);
#20290=ORIENTED_EDGE('',*,*,#14997,.T.);
#20291=ORIENTED_EDGE('',*,*,#15005,.T.);
#20292=ORIENTED_EDGE('',*,*,#14988,.T.);
#20293=ORIENTED_EDGE('',*,*,#15006,.T.);
#20294=ORIENTED_EDGE('',*,*,#15007,.T.);
#20295=ORIENTED_EDGE('',*,*,#15008,.T.);
#20296=ORIENTED_EDGE('',*,*,#15006,.F.);
#20297=ORIENTED_EDGE('',*,*,#15009,.T.);
#20298=ORIENTED_EDGE('',*,*,#15010,.T.);
#20299=ORIENTED_EDGE('',*,*,#15011,.T.);
#20300=ORIENTED_EDGE('',*,*,#15012,.F.);
#20301=ORIENTED_EDGE('',*,*,#15013,.T.);
#20302=ORIENTED_EDGE('',*,*,#15007,.F.);
#20303=ORIENTED_EDGE('',*,*,#15008,.F.);
#20304=ORIENTED_EDGE('',*,*,#15013,.F.);
#20305=ORIENTED_EDGE('',*,*,#15014,.T.);
#20306=ORIENTED_EDGE('',*,*,#15015,.T.);
#20307=ORIENTED_EDGE('',*,*,#15016,.F.);
#20308=ORIENTED_EDGE('',*,*,#15015,.F.);
#20309=ORIENTED_EDGE('',*,*,#15011,.F.);
#20310=ORIENTED_EDGE('',*,*,#15010,.F.);
#20311=ORIENTED_EDGE('',*,*,#15009,.F.);
#20312=ORIENTED_EDGE('',*,*,#15017,.T.);
#20313=ORIENTED_EDGE('',*,*,#15012,.T.);
#20314=ORIENTED_EDGE('',*,*,#15017,.F.);
#20315=ORIENTED_EDGE('',*,*,#14984,.T.);
#20316=ORIENTED_EDGE('',*,*,#14987,.F.);
#20317=ORIENTED_EDGE('',*,*,#15003,.F.);
#20318=ORIENTED_EDGE('',*,*,#15000,.T.);
#20319=ORIENTED_EDGE('',*,*,#14998,.T.);
#20320=ORIENTED_EDGE('',*,*,#15004,.F.);
#20321=ORIENTED_EDGE('',*,*,#14989,.F.);
#20322=ORIENTED_EDGE('',*,*,#15005,.F.);
#20323=ORIENTED_EDGE('',*,*,#14996,.T.);
#20324=ORIENTED_EDGE('',*,*,#15002,.F.);
#20325=ORIENTED_EDGE('',*,*,#15014,.F.);
#20326=ORIENTED_EDGE('',*,*,#15016,.T.);
#20327=ORIENTED_EDGE('',*,*,#15018,.T.);
#20328=ORIENTED_EDGE('',*,*,#15019,.F.);
#20329=ORIENTED_EDGE('',*,*,#15018,.F.);
#20330=ORIENTED_EDGE('',*,*,#15020,.F.);
#20331=ORIENTED_EDGE('',*,*,#15019,.T.);
#20332=ORIENTED_EDGE('',*,*,#14982,.F.);
#20333=ORIENTED_EDGE('',*,*,#15021,.T.);
#20334=ORIENTED_EDGE('',*,*,#15020,.T.);
#20335=ORIENTED_EDGE('',*,*,#15021,.F.);
#20336=ORIENTED_EDGE('',*,*,#15001,.F.);
#20337=ORIENTED_EDGE('',*,*,#15022,.T.);
#20338=ORIENTED_EDGE('',*,*,#14980,.T.);
#20339=ORIENTED_EDGE('',*,*,#15022,.F.);
#25340=CONICAL_SURFACE('',#27796,1.08,0.785398163397454);
#25341=CONICAL_SURFACE('',#27812,3.0525,0.785398163397448);
#25342=CONICAL_SURFACE('',#27816,7.4,0.785398163397448);
#25343=CONICAL_SURFACE('',#27817,7.4,0.785398163397448);
#25916=ADVANCED_FACE('',(#3103),#280,.T.);
#25917=ADVANCED_FACE('',(#3104,#868,#869,#870),#723,.T.);
#25918=ADVANCED_FACE('',(#3105,#871),#724,.F.);
#25919=ADVANCED_FACE('',(#3106),#281,.T.);
#25920=ADVANCED_FACE('',(#3107),#25340,.F.);
#25921=ADVANCED_FACE('',(#3108),#725,.F.);
#25922=ADVANCED_FACE('',(#3109,#872),#1911,.T.);
#25923=ADVANCED_FACE('',(#3110),#282,.T.);
#25924=ADVANCED_FACE('',(#3111),#283,.T.);
#25925=ADVANCED_FACE('',(#3112),#284,.T.);
#25926=ADVANCED_FACE('',(#3113),#726,.F.);
#25927=ADVANCED_FACE('',(#3114,#873),#727,.F.);
#25928=ADVANCED_FACE('',(#3115),#285,.T.);
#25929=ADVANCED_FACE('',(#3116),#1912,.F.);
#25930=ADVANCED_FACE('',(#3117),#1913,.F.);
#25931=ADVANCED_FACE('',(#3118),#1914,.T.);
#25932=ADVANCED_FACE('',(#3119),#25341,.F.);
#25933=ADVANCED_FACE('',(#3120,#874),#1915,.T.);
#25934=ADVANCED_FACE('',(#3121),#25342,.T.);
#25935=ADVANCED_FACE('',(#3122),#25343,.T.);
#26882=CLOSED_SHELL('',(#25916,#25917,#25918,#25919,#25920,#25921,#25922,
#25923,#25924,#25925,#25926,#25927,#25928,#25929,#25930,#25931,#25932,#25933,
#25934,#25935));
#27791=AXIS2_PLACEMENT_3D('',#59483,#31065,#31066);
#27792=AXIS2_PLACEMENT_3D('',#59763,#31068,#31069);
#27793=AXIS2_PLACEMENT_3D('',#59765,#31070,#31071);
#27794=AXIS2_PLACEMENT_3D('',#59768,#31073,#31074);
#27795=AXIS2_PLACEMENT_3D('',#59883,#31075,#31076);
#27796=AXIS2_PLACEMENT_3D('',#60182,#31081,#31082);
#27797=AXIS2_PLACEMENT_3D('',#60184,#31083,#31084);
#27798=AXIS2_PLACEMENT_3D('',#60187,#31086,#31087);
#27799=AXIS2_PLACEMENT_3D('',#60188,#31088,#31089);
#27800=AXIS2_PLACEMENT_3D('',#60207,#31090,#31091);
#27801=AXIS2_PLACEMENT_3D('',#60224,#31092,#31093);
#27802=AXIS2_PLACEMENT_3D('',#60226,#31095,#31096);
#27803=AXIS2_PLACEMENT_3D('',#60227,#31097,#31098);
#27804=AXIS2_PLACEMENT_3D('',#60229,#31099,#31100);
#27805=AXIS2_PLACEMENT_3D('',#60532,#31102,#31103);
#27806=AXIS2_PLACEMENT_3D('',#60593,#31105,#31106);
#27807=AXIS2_PLACEMENT_3D('',#60595,#31107,#31108);
#27808=AXIS2_PLACEMENT_3D('',#60598,#31110,#31111);
#27809=AXIS2_PLACEMENT_3D('',#60832,#31113,#31114);
#27810=AXIS2_PLACEMENT_3D('',#60833,#31115,#31116);
#27811=AXIS2_PLACEMENT_3D('',#60834,#31117,#31118);
#27812=AXIS2_PLACEMENT_3D('',#60835,#31119,#31120);
#27813=AXIS2_PLACEMENT_3D('',#60838,#31122,#31123);
#27814=AXIS2_PLACEMENT_3D('',#60839,#31124,#31125);
#27815=AXIS2_PLACEMENT_3D('',#60841,#31126,#31127);
#27816=AXIS2_PLACEMENT_3D('',#60842,#31128,#31129);
#27817=AXIS2_PLACEMENT_3D('',#60844,#31131,#31132);
#31065=DIRECTION('axis',(0.,0.,1.));
#31066=DIRECTION('refdir',(1.,0.,0.));
#31067=DIRECTION('',(0.545504242983751,0.,0.838108060387636));
#31068=DIRECTION('center_axis',(0.,-1.,0.));
#31069=DIRECTION('ref_axis',(1.,0.,0.));
#31070=DIRECTION('center_axis',(0.,-1.,0.));
#31071=DIRECTION('ref_axis',(1.,0.,0.));
#31072=DIRECTION('',(0.,1.,0.));
#31073=DIRECTION('center_axis',(0.,-1.,0.));
#31074=DIRECTION('ref_axis',(1.,0.,0.));
#31075=DIRECTION('center_axis',(-0.342020143325669,0.,0.939692620785908));
#31076=DIRECTION('ref_axis',(0.939692620785909,0.,0.342020143325668));
#31077=DIRECTION('',(-0.342020143325669,0.,0.939692620785908));
#31078=DIRECTION('',(0.342020143325669,0.,-0.939692620785908));
#31079=DIRECTION('',(-0.342020143325669,0.,0.939692620785908));
#31080=DIRECTION('',(0.956605970831105,0.,-0.291384653971824));
#31081=DIRECTION('center_axis',(0.,-1.,0.));
#31082=DIRECTION('ref_axis',(1.,0.,0.));
#31083=DIRECTION('center_axis',(0.,-1.,0.));
#31084=DIRECTION('ref_axis',(1.,0.,0.));
#31085=DIRECTION('',(0.707106781186552,0.707106781186543,8.65956056235498E-17));
#31086=DIRECTION('center_axis',(0.,1.,0.));
#31087=DIRECTION('ref_axis',(1.,0.,0.));
#31088=DIRECTION('center_axis',(0.,-1.,0.));
#31089=DIRECTION('ref_axis',(1.,0.,0.));
#31090=DIRECTION('center_axis',(0.,-1.,0.));
#31091=DIRECTION('ref_axis',(1.,0.,0.));
#31092=DIRECTION('center_axis',(0.,-1.,0.));
#31093=DIRECTION('ref_axis',(1.,0.,0.));
#31094=DIRECTION('',(0.,-1.,0.));
#31095=DIRECTION('center_axis',(0.,-1.,0.));
#31096=DIRECTION('ref_axis',(1.,0.,0.));
#31097=DIRECTION('center_axis',(0.,-1.,0.));
#31098=DIRECTION('ref_axis',(0.,0.,-1.));
#31099=DIRECTION('center_axis',(0.,-1.,0.));
#31100=DIRECTION('ref_axis',(1.,0.,0.));
#31101=DIRECTION('',(0.657622941203057,-0.70669776106396,0.260979581022399));
#31102=DIRECTION('center_axis',(-0.939692620785908,0.,-0.342020143325669));
#31103=DIRECTION('ref_axis',(-0.342020143325669,0.,0.939692620785908));
#31104=DIRECTION('',(-0.939692620785908,0.,-0.342020143325669));
#31105=DIRECTION('center_axis',(0.,-1.,0.));
#31106=DIRECTION('ref_axis',(1.,0.,0.));
#31107=DIRECTION('center_axis',(0.,-1.,0.));
#31108=DIRECTION('ref_axis',(1.,0.,0.));
#31109=DIRECTION('',(0.,1.,0.));
#31110=DIRECTION('center_axis',(0.,-1.,0.));
#31111=DIRECTION('ref_axis',(1.,0.,0.));
#31112=DIRECTION('',(-0.87991994563834,0.,0.475121973042524));
#31113=DIRECTION('center_axis',(0.,1.,0.));
#31114=DIRECTION('ref_axis',(0.,0.,1.));
#31115=DIRECTION('center_axis',(0.,1.,0.));
#31116=DIRECTION('ref_axis',(0.,0.,1.));
#31117=DIRECTION('center_axis',(0.,1.,0.));
#31118=DIRECTION('ref_axis',(0.,0.,1.));
#31119=DIRECTION('center_axis',(0.,1.,0.));
#31120=DIRECTION('ref_axis',(1.,0.,0.));
#31121=DIRECTION('',(-0.707106781186547,0.707106781186547,-8.65956056235493E-17));
#31122=DIRECTION('center_axis',(0.,-1.,0.));
#31123=DIRECTION('ref_axis',(1.,0.,0.));
#31124=DIRECTION('center_axis',(0.,1.,0.));
#31125=DIRECTION('ref_axis',(0.,0.,1.));
#31126=DIRECTION('center_axis',(0.,-1.,0.));
#31127=DIRECTION('ref_axis',(1.,0.,0.));
#31128=DIRECTION('center_axis',(0.,-1.,0.));
#31129=DIRECTION('ref_axis',(1.,0.,0.));
#31130=DIRECTION('',(0.707106781186548,0.707106781186548,8.65956056235493E-17));
#31131=DIRECTION('center_axis',(0.,1.,0.));
#31132=DIRECTION('ref_axis',(1.,0.,0.));
#31133=DIRECTION('',(-0.707106781186548,0.707106781186548,-8.65956056235493E-17));
#59483=CARTESIAN_POINT('',(0.,0.,0.));
#59484=CARTESIAN_POINT('Ctrl Pts',(9.74287700479826,-21.5,70.5125025877322));
#59485=CARTESIAN_POINT('Ctrl Pts',(9.74287700479826,-21.656214196966,70.5125025877322));
#59486=CARTESIAN_POINT('Ctrl Pts',(9.77861943028971,-21.9803373691276,70.5144059476976));
#59487=CARTESIAN_POINT('Ctrl Pts',(9.92068473931345,-22.3731848943024,70.5242594183206));
#59488=CARTESIAN_POINT('Ctrl Pts',(10.083942330172,-22.6596849246672,70.5396163501376));
#59489=CARTESIAN_POINT('Ctrl Pts',(10.2764424102782,-22.9226724124575,70.5614144955755));
#59490=CARTESIAN_POINT('Ctrl Pts',(10.5505406389766,-23.1948597886741,70.600128983041));
#59491=CARTESIAN_POINT('Ctrl Pts',(10.8954109293732,-23.4174824644433,70.6667169758025));
#59492=CARTESIAN_POINT('Ctrl Pts',(11.1554284786727,-23.5274756480171,70.7298614280393));
#59493=CARTESIAN_POINT('Ctrl Pts',(11.2883532161314,-23.5711895983197,70.7654371551999));
#59494=CARTESIAN_POINT('Ctrl Pts',(11.3646737922248,-23.5926452515457,70.7868530255724));
#59495=CARTESIAN_POINT('Ctrl Pts',(11.5562073871596,-23.6406588378193,70.8422231900863));
#59496=CARTESIAN_POINT('Ctrl Pts',(11.7658252370385,-23.664271882774,70.9111982308898));
#59497=CARTESIAN_POINT('Ctrl Pts',(12.0578852179822,-23.6557172786385,71.0201457155622));
#59498=CARTESIAN_POINT('Ctrl Pts',(12.2208094014591,-23.6319919884316,71.0867018338967));
#59499=CARTESIAN_POINT('Ctrl Pts',(12.3543904463612,-23.5975235527391,71.1456250307213));
#59500=CARTESIAN_POINT('Ctrl Pts',(12.4027779159087,-23.5839664204326,71.167268720936));
#59501=CARTESIAN_POINT('Ctrl Pts',(12.4866718330575,-23.5575942766802,71.2055992342487));
#59502=CARTESIAN_POINT('Ctrl Pts',(12.6510577647346,-23.4940583870137,71.2838949455475));
#59503=CARTESIAN_POINT('Ctrl Pts',(12.8719512966863,-23.3748625900797,71.3976849620357));
#59504=CARTESIAN_POINT('Ctrl Pts',(13.1084649034627,-23.1892327479386,71.5314239215564));
#59505=CARTESIAN_POINT('Ctrl Pts',(13.3051919767247,-22.9780992092235,71.6514654851331));
#59506=CARTESIAN_POINT('Ctrl Pts',(13.4763850760173,-22.7304324210399,71.7627534820972));
#59507=CARTESIAN_POINT('Ctrl Pts',(13.6168015105668,-22.4461912796831,71.8592569555153));
#59508=CARTESIAN_POINT('Ctrl Pts',(13.709674381118,-22.1641725337909,71.9258725275639));
#59509=CARTESIAN_POINT('Ctrl Pts',(13.7535308851104,-21.9512225876456,71.9580350138515));
#59510=CARTESIAN_POINT('Ctrl Pts',(13.7979233224896,-21.6302708884948,71.9909065809688));
#59511=CARTESIAN_POINT('Ctrl Pts',(13.7985524061519,-21.2911597238678,71.9912918069344));
#59512=CARTESIAN_POINT('Ctrl Pts',(13.7183983186692,-20.8609704899414,71.932093483098));
#59513=CARTESIAN_POINT('Ctrl Pts',(13.6166712998014,-20.5540190040535,71.8591758531238));
#59514=CARTESIAN_POINT('Ctrl Pts',(13.4764722169006,-20.2695559196014,71.7628122981255));
#59515=CARTESIAN_POINT('Ctrl Pts',(13.30479452339,-20.0214367560947,71.6512132027746));
#59516=CARTESIAN_POINT('Ctrl Pts',(13.108633737568,-19.8110230421895,71.5315418245281));
#59517=CARTESIAN_POINT('Ctrl Pts',(12.9112681237482,-19.656071853345,71.4199434952884));
#59518=CARTESIAN_POINT('Ctrl Pts',(12.6535693601998,-19.5026800844597,71.2842239697829));
#59519=CARTESIAN_POINT('Ctrl Pts',(12.3693061289729,-19.3924814953289,71.1481752603989));
#59520=CARTESIAN_POINT('Ctrl Pts',(12.0216107241993,-19.338052834614,71.005036372742));
#59521=CARTESIAN_POINT('Ctrl Pts',(11.6310650689274,-19.3376578948939,70.8625951386498));
#59522=CARTESIAN_POINT('Ctrl Pts',(11.1091117678361,-19.4569229967783,70.7097325311002));
#59523=CARTESIAN_POINT('Ctrl Pts',(10.5875357806613,-19.7677773346453,70.6053394071194));
#59524=CARTESIAN_POINT('Ctrl Pts',(10.3040349212154,-20.0501861211832,70.5653346387674));
#59525=CARTESIAN_POINT('Ctrl Pts',(10.1066531997307,-20.305521444769,70.5419005952258));
#59526=CARTESIAN_POINT('Ctrl Pts',(9.93487527850697,-20.5875814819759,70.5252370307246));
#59527=CARTESIAN_POINT('Ctrl Pts',(9.77867795084425,-21.0196494588534,70.5144182338898));
#59528=CARTESIAN_POINT('Ctrl Pts',(9.74287700479826,-21.3437858030339,70.5125025877322));
#59529=CARTESIAN_POINT('Ctrl Pts',(9.74287700479826,-21.5,70.5125025877322));
#59530=CARTESIAN_POINT('Ctrl Pts',(9.77566129268524,-21.5,70.5628720876684));
#59531=CARTESIAN_POINT('Ctrl Pts',(9.77566129268524,-21.6534741316411,70.5628720876684));
#59532=CARTESIAN_POINT('Ctrl Pts',(9.81099168028511,-21.9719192919697,70.5650519513878));
#59533=CARTESIAN_POINT('Ctrl Pts',(9.95117347313436,-22.3572458209345,70.5758665902743));
#59534=CARTESIAN_POINT('Ctrl Pts',(10.1118579963003,-22.6376328078247,70.5920838302201));
#59535=CARTESIAN_POINT('Ctrl Pts',(10.3009739420384,-22.8945540804684,70.6146705888467));
#59536=CARTESIAN_POINT('Ctrl Pts',(10.5695498424849,-23.1596691288769,70.6540368613604));
#59537=CARTESIAN_POINT('Ctrl Pts',(10.9060823062057,-23.3756123556826,70.7203264012894));
#59538=CARTESIAN_POINT('Ctrl Pts',(11.1590889733824,-23.4820149939127,70.7824430077388));
#59539=CARTESIAN_POINT('Ctrl Pts',(11.2883004649771,-23.5242631039492,70.8172953874664));
#59540=CARTESIAN_POINT('Ctrl Pts',(11.3624559776584,-23.5449889102041,70.838237600039));
#59541=CARTESIAN_POINT('Ctrl Pts',(11.5485093899437,-23.5913547053039,70.8923250019762));
#59542=CARTESIAN_POINT('Ctrl Pts',(11.7519243617111,-23.6141195484566,70.959414244256));
#59543=CARTESIAN_POINT('Ctrl Pts',(12.0354296368004,-23.6058714701567,71.0651137905936));
#59544=CARTESIAN_POINT('Ctrl Pts',(12.193665998477,-23.5829845184256,71.1295980617617));
#59545=CARTESIAN_POINT('Ctrl Pts',(12.3235593632531,-23.5497000132635,71.1866674340606));
#59546=CARTESIAN_POINT('Ctrl Pts',(12.3706227200289,-23.5366057407861,71.2076295818757));
#59547=CARTESIAN_POINT('Ctrl Pts',(12.4522536209234,-23.5111271728441,71.2447520528871));
#59548=CARTESIAN_POINT('Ctrl Pts',(12.6123491063975,-23.4497024850363,71.3205844405804));
#59549=CARTESIAN_POINT('Ctrl Pts',(12.8279339405974,-23.3343024876679,71.4308465647072));
#59550=CARTESIAN_POINT('Ctrl Pts',(13.0595565632642,-23.1540884860638,71.5606184977724));
#59551=CARTESIAN_POINT('Ctrl Pts',(13.2528809724359,-22.9485568459442,71.6772866701138));
#59552=CARTESIAN_POINT('Ctrl Pts',(13.4216736669167,-22.7068367362783,71.785623374226));
#59553=CARTESIAN_POINT('Ctrl Pts',(13.5605733827612,-22.4287379648088,71.8797176190141));
#59554=CARTESIAN_POINT('Ctrl Pts',(13.6526950213329,-22.1522500472725,71.9447564871425));
#59555=CARTESIAN_POINT('Ctrl Pts',(13.6962620308405,-21.9432179955209,71.976180116676));
#59556=CARTESIAN_POINT('Ctrl Pts',(13.740391047937,-21.6280318714313,72.0083066859187));
#59557=CARTESIAN_POINT('Ctrl Pts',(13.7410087312265,-21.2947483967792,72.0086804998937));
#59558=CARTESIAN_POINT('Ctrl Pts',(13.6613448700357,-20.8723984338637,71.9508289201672));
#59559=CARTESIAN_POINT('Ctrl Pts',(13.5604453574354,-20.5714697858188,71.8796387836749));
#59560=CARTESIAN_POINT('Ctrl Pts',(13.4217594678946,-20.2931514421549,71.7856804754748));
#59561=CARTESIAN_POINT('Ctrl Pts',(13.2524898178296,-20.0509908996673,71.6770412767522));
#59562=CARTESIAN_POINT('Ctrl Pts',(13.0597225605965,-19.8461608875654,71.5607328512164));
#59563=CARTESIAN_POINT('Ctrl Pts',(12.8664408368138,-19.695729310016,71.4524457223248));
#59564=CARTESIAN_POINT('Ctrl Pts',(12.6147312978391,-19.5471004559845,71.320886585664));
#59565=CARTESIAN_POINT('Ctrl Pts',(12.3379146864166,-19.4406307679279,71.1891521581768));
#59566=CARTESIAN_POINT('Ctrl Pts',(12.0001882251287,-19.3881193545174,71.0504767635001));
#59567=CARTESIAN_POINT('Ctrl Pts',(11.621154655613,-19.3877604898925,70.9122445590948));
#59568=CARTESIAN_POINT('Ctrl Pts',(11.1144403261534,-19.5027306944885,70.7630434730559));
#59569=CARTESIAN_POINT('Ctrl Pts',(10.6058218204276,-19.8039173677725,70.659337688344));
#59570=CARTESIAN_POINT('Ctrl Pts',(10.3280066988785,-20.0790135058352,70.6186547075878));
#59571=CARTESIAN_POINT('Ctrl Pts',(10.134197724029,-20.3283456136423,70.5944789024564));
#59572=CARTESIAN_POINT('Ctrl Pts',(9.96517644530526,-20.6042709357116,70.5769404654071));
#59573=CARTESIAN_POINT('Ctrl Pts',(9.8110491734264,-21.0280688465375,70.5650642368601));
#59574=CARTESIAN_POINT('Ctrl Pts',(9.77566129268524,-21.3465258683589,70.5628720876684));
#59575=CARTESIAN_POINT('Ctrl Pts',(9.77566129268524,-21.5,70.5628720876684));
#59576=CARTESIAN_POINT('Ctrl Pts',(9.80844558057222,-21.5,70.6132415876045));
#59577=CARTESIAN_POINT('Ctrl Pts',(9.80844558057222,-21.6507340663161,70.6132415876045));
#59578=CARTESIAN_POINT('Ctrl Pts',(9.84336393028051,-21.9635012148119,70.615697955078));
#59579=CARTESIAN_POINT('Ctrl Pts',(9.98166220695528,-22.3413067475665,70.6274737622279));
#59580=CARTESIAN_POINT('Ctrl Pts',(10.1397736624286,-22.6155806909822,70.6445513103028));
#59581=CARTESIAN_POINT('Ctrl Pts',(10.3255054737985,-22.8664357484793,70.667926682118));
#59582=CARTESIAN_POINT('Ctrl Pts',(10.5885590459932,-23.1244784690798,70.7079447396797));
#59583=CARTESIAN_POINT('Ctrl Pts',(10.9167536830382,-23.333742246922,70.7739358267763));
#59584=CARTESIAN_POINT('Ctrl Pts',(11.1627494680922,-23.4365543398082,70.8350245874384));
#59585=CARTESIAN_POINT('Ctrl Pts',(11.2882477138228,-23.4773366095787,70.869153619733));
#59586=CARTESIAN_POINT('Ctrl Pts',(11.360238163092,-23.4973325688625,70.8896221745056));
#59587=CARTESIAN_POINT('Ctrl Pts',(11.5408113927277,-23.5420505727884,70.9424268138662));
#59588=CARTESIAN_POINT('Ctrl Pts',(11.7380234863837,-23.5639672141393,71.0076302576221));
#59589=CARTESIAN_POINT('Ctrl Pts',(12.0129740556185,-23.5560256616749,71.1100818656249));
#59590=CARTESIAN_POINT('Ctrl Pts',(12.1665225954948,-23.5339770484196,71.1724942896266));
#59591=CARTESIAN_POINT('Ctrl Pts',(12.2927282801449,-23.5018764737878,71.2277098374));
#59592=CARTESIAN_POINT('Ctrl Pts',(12.3384675241492,-23.4892450611396,71.2479904428155));
#59593=CARTESIAN_POINT('Ctrl Pts',(12.4178354087892,-23.4646600690079,71.2839048715255));
#59594=CARTESIAN_POINT('Ctrl Pts',(12.5736404480604,-23.4053465830588,71.3572739356134));
#59595=CARTESIAN_POINT('Ctrl Pts',(12.7839165845085,-23.2937423852561,71.4640081673788));
#59596=CARTESIAN_POINT('Ctrl Pts',(13.0106482230657,-23.118944224189,71.5898130739885));
#59597=CARTESIAN_POINT('Ctrl Pts',(13.2005699681471,-22.919014482665,71.7031078550945));
#59598=CARTESIAN_POINT('Ctrl Pts',(13.366962257816,-22.6832410515167,71.8084932663548));
#59599=CARTESIAN_POINT('Ctrl Pts',(13.5043452549556,-22.4112846499345,71.9001782825129));
#59600=CARTESIAN_POINT('Ctrl Pts',(13.5957156615478,-22.1403275607541,71.9636404467212));
#59601=CARTESIAN_POINT('Ctrl Pts',(13.6389931765705,-21.9352134033963,71.9943252195005));
#59602=CARTESIAN_POINT('Ctrl Pts',(13.6828587733844,-21.6257928543678,72.0257067908687));
#59603=CARTESIAN_POINT('Ctrl Pts',(13.6834650563012,-21.2983370696906,72.0260691928531));
#59604=CARTESIAN_POINT('Ctrl Pts',(13.6042914214022,-20.883826377786,71.9695643572363));
#59605=CARTESIAN_POINT('Ctrl Pts',(13.5042194150694,-20.588920567584,71.900101714226));
#59606=CARTESIAN_POINT('Ctrl Pts',(13.3670467188885,-20.3167469647085,71.808548652824));
#59607=CARTESIAN_POINT('Ctrl Pts',(13.2001851122691,-20.0805450432399,71.7028693507298));
#59608=CARTESIAN_POINT('Ctrl Pts',(13.0108113836249,-19.8812987329413,71.5899238779046));
#59609=CARTESIAN_POINT('Ctrl Pts',(12.8216135498794,-19.7353867666869,71.4849479493612));
#59610=CARTESIAN_POINT('Ctrl Pts',(12.5758932354784,-19.5915208275092,71.3575492015453));
#59611=CARTESIAN_POINT('Ctrl Pts',(12.3065232438603,-19.4887800405268,71.2301290559547));
#59612=CARTESIAN_POINT('Ctrl Pts',(11.9787657260582,-19.4381858744207,71.0959171542583));
#59613=CARTESIAN_POINT('Ctrl Pts',(11.6112442422986,-19.4378630848911,70.9618939795399));
#59614=CARTESIAN_POINT('Ctrl Pts',(11.1197688844706,-19.5485383921987,70.8163544150116));
#59615=CARTESIAN_POINT('Ctrl Pts',(10.624107860194,-19.8400574008998,70.7133359695685));
#59616=CARTESIAN_POINT('Ctrl Pts',(10.3519784765416,-20.1078408904872,70.6719747764082));
#59617=CARTESIAN_POINT('Ctrl Pts',(10.1617422483273,-20.3511697825156,70.6470572096869));
#59618=CARTESIAN_POINT('Ctrl Pts',(9.99547761210354,-20.6209603894473,70.6286439000895));
#59619=CARTESIAN_POINT('Ctrl Pts',(9.84342039600855,-21.0364882342215,70.6157102398303));
#59620=CARTESIAN_POINT('Ctrl Pts',(9.80844558057223,-21.3492659336839,70.6132415876045));
#59621=CARTESIAN_POINT('Ctrl Pts',(9.80844558057223,-21.5,70.6132415876045));
#59622=CARTESIAN_POINT('Ctrl Pts',(9.8412298684592,-21.5,70.6636110875407));
#59623=CARTESIAN_POINT('Ctrl Pts',(9.8412298684592,-21.6479940009911,70.6636110875407));
#59624=CARTESIAN_POINT('Ctrl Pts',(9.87573618027591,-21.9550831376541,70.6663439587683));
#59625=CARTESIAN_POINT('Ctrl Pts',(10.0121509407762,-22.3253676741985,70.6790809341815));
#59626=CARTESIAN_POINT('Ctrl Pts',(10.1676893285569,-22.5935285741397,70.6970187903853));
#59627=CARTESIAN_POINT('Ctrl Pts',(10.3500370055587,-22.8383174164902,70.7211827753892));
#59628=CARTESIAN_POINT('Ctrl Pts',(10.6075682495015,-23.0892878092826,70.7618526179991));
#59629=CARTESIAN_POINT('Ctrl Pts',(10.9274250598707,-23.2918721381614,70.8275452522632));
#59630=CARTESIAN_POINT('Ctrl Pts',(11.1664099628019,-23.3910936857038,70.8876061671379));
#59631=CARTESIAN_POINT('Ctrl Pts',(11.2881949626684,-23.4304101152083,70.9210118519996));
#59632=CARTESIAN_POINT('Ctrl Pts',(11.3580203485256,-23.4496762275209,70.9410067489722));
#59633=CARTESIAN_POINT('Ctrl Pts',(11.5331133955118,-23.4927464402729,70.9925286257561));
#59634=CARTESIAN_POINT('Ctrl Pts',(11.7241226110564,-23.513814879822,71.0558462709882));
#59635=CARTESIAN_POINT('Ctrl Pts',(11.9905184744366,-23.5061798531931,71.1550499406563));
#59636=CARTESIAN_POINT('Ctrl Pts',(12.1393791925127,-23.4849695784135,71.2153905174916));
#59637=CARTESIAN_POINT('Ctrl Pts',(12.2618971970367,-23.4540529343121,71.2687522407393));
#59638=CARTESIAN_POINT('Ctrl Pts',(12.3063123282695,-23.4418843814931,71.2883513037553));
#59639=CARTESIAN_POINT('Ctrl Pts',(12.3834171966551,-23.4181929651718,71.3230576901639));
#59640=CARTESIAN_POINT('Ctrl Pts',(12.5349317897233,-23.3609906810814,71.3939634306464));
#59641=CARTESIAN_POINT('Ctrl Pts',(12.7398992284196,-23.2531822828443,71.4971697700503));
#59642=CARTESIAN_POINT('Ctrl Pts',(12.9617398828672,-23.0837999623142,71.6190076502045));
#59643=CARTESIAN_POINT('Ctrl Pts',(13.1482589638583,-22.8894721193857,71.7289290400752));
#59644=CARTESIAN_POINT('Ctrl Pts',(13.3122508487154,-22.6596453667551,71.8313631584836));
#59645=CARTESIAN_POINT('Ctrl Pts',(13.4481171271501,-22.3938313350602,71.9206389460116));
#59646=CARTESIAN_POINT('Ctrl Pts',(13.5387363017626,-22.1284050742357,71.9825244062999));
#59647=CARTESIAN_POINT('Ctrl Pts',(13.5817243223006,-21.9272088112716,72.012470322325));
#59648=CARTESIAN_POINT('Ctrl Pts',(13.6253264988318,-21.6235538373044,72.0431068958186));
#59649=CARTESIAN_POINT('Ctrl Pts',(13.6259213813758,-21.301925742602,72.0434578858125));
#59650=CARTESIAN_POINT('Ctrl Pts',(13.5472379727687,-20.8952543217083,71.9882997943055));
#59651=CARTESIAN_POINT('Ctrl Pts',(13.4479934727035,-20.6063713493493,71.9205646447771));
#59652=CARTESIAN_POINT('Ctrl Pts',(13.3123339698825,-20.340342487262,71.8314168301733));
#59653=CARTESIAN_POINT('Ctrl Pts',(13.1478804067087,-20.1100991868126,71.7286974247074));
#59654=CARTESIAN_POINT('Ctrl Pts',(12.9619002066534,-19.9164365783173,71.6191149045929));
#59655=CARTESIAN_POINT('Ctrl Pts',(12.7767862629449,-19.7750442233578,71.5174501763976));
#59656=CARTESIAN_POINT('Ctrl Pts',(12.5370551731176,-19.6359411990339,71.3942118174265));
#59657=CARTESIAN_POINT('Ctrl Pts',(12.275131801304,-19.5369293131258,71.2711059537325));
#59658=CARTESIAN_POINT('Ctrl Pts',(11.9573432269876,-19.4882523943241,71.1413575450164));
#59659=CARTESIAN_POINT('Ctrl Pts',(11.6013338289841,-19.4879656798897,71.011543399985));
#59660=CARTESIAN_POINT('Ctrl Pts',(11.1250974427879,-19.5943460899089,70.8696653569674));
#59661=CARTESIAN_POINT('Ctrl Pts',(10.6423938999603,-19.876197434027,70.7673342507931));
#59662=CARTESIAN_POINT('Ctrl Pts',(10.3759502542046,-20.1366682751392,70.7252948452286));
#59663=CARTESIAN_POINT('Ctrl Pts',(10.1892867726256,-20.3739939513888,70.6996355169175));
#59664=CARTESIAN_POINT('Ctrl Pts',(10.0257787789018,-20.637649843183,70.6803473347719));
#59665=CARTESIAN_POINT('Ctrl Pts',(9.8757916185907,-21.0449076219056,70.6663562428006));
#59666=CARTESIAN_POINT('Ctrl Pts',(9.84122986845921,-21.3520059990089,70.6636110875407));
#59667=CARTESIAN_POINT('Ctrl Pts',(9.84122986845921,-21.5,70.6636110875407));
#59668=CARTESIAN_POINT('',(9.74287700479826,-21.5,70.5125025877322));
#59669=CARTESIAN_POINT('',(9.8412298684592,-21.5,70.6636110875407));
#59670=CARTESIAN_POINT('',(9.74287700479826,-21.5,70.5125025877322));
#59671=CARTESIAN_POINT('Ctrl Pts',(9.8412298684592,-21.5,70.6636110875407));
#59672=CARTESIAN_POINT('Ctrl Pts',(9.8412298684592,-21.6479940009911,70.6636110875407));
#59673=CARTESIAN_POINT('Ctrl Pts',(9.87573618027591,-21.9550831376541,70.6663439587683));
#59674=CARTESIAN_POINT('Ctrl Pts',(10.0121509407762,-22.3253676741985,70.6790809341815));
#59675=CARTESIAN_POINT('Ctrl Pts',(10.1676893285569,-22.5935285741397,70.6970187903853));
#59676=CARTESIAN_POINT('Ctrl Pts',(10.3500370055587,-22.8383174164902,70.7211827753892));
#59677=CARTESIAN_POINT('Ctrl Pts',(10.6075682495015,-23.0892878092826,70.7618526179991));
#59678=CARTESIAN_POINT('Ctrl Pts',(10.9274250598707,-23.2918721381614,70.8275452522632));
#59679=CARTESIAN_POINT('Ctrl Pts',(11.1664099628019,-23.3910936857038,70.8876061671379));
#59680=CARTESIAN_POINT('Ctrl Pts',(11.2881949626684,-23.4304101152083,70.9210118519996));
#59681=CARTESIAN_POINT('Ctrl Pts',(11.3580203485256,-23.4496762275209,70.9410067489722));
#59682=CARTESIAN_POINT('Ctrl Pts',(11.5331133955118,-23.4927464402729,70.9925286257561));
#59683=CARTESIAN_POINT('Ctrl Pts',(11.7241226110564,-23.513814879822,71.0558462709882));
#59684=CARTESIAN_POINT('Ctrl Pts',(11.9905184744366,-23.5061798531931,71.1550499406563));
#59685=CARTESIAN_POINT('Ctrl Pts',(12.1393791925127,-23.4849695784135,71.2153905174916));
#59686=CARTESIAN_POINT('Ctrl Pts',(12.2618971970367,-23.4540529343121,71.2687522407393));
#59687=CARTESIAN_POINT('Ctrl Pts',(12.3063123282695,-23.4418843814931,71.2883513037553));
#59688=CARTESIAN_POINT('Ctrl Pts',(12.3834171966551,-23.4181929651718,71.3230576901639));
#59689=CARTESIAN_POINT('Ctrl Pts',(12.5349317897233,-23.3609906810814,71.3939634306464));
#59690=CARTESIAN_POINT('Ctrl Pts',(12.7398992284196,-23.2531822828443,71.4971697700503));
#59691=CARTESIAN_POINT('Ctrl Pts',(12.9617398828672,-23.0837999623142,71.6190076502045));
#59692=CARTESIAN_POINT('Ctrl Pts',(13.1482589638583,-22.8894721193857,71.7289290400752));
#59693=CARTESIAN_POINT('Ctrl Pts',(13.3122508487154,-22.6596453667551,71.8313631584836));
#59694=CARTESIAN_POINT('Ctrl Pts',(13.4481171271501,-22.3938313350602,71.9206389460116));
#59695=CARTESIAN_POINT('Ctrl Pts',(13.5387363017626,-22.1284050742357,71.9825244062999));
#59696=CARTESIAN_POINT('Ctrl Pts',(13.5817243223006,-21.9272088112716,72.012470322325));
#59697=CARTESIAN_POINT('Ctrl Pts',(13.6253264988318,-21.6235538373044,72.0431068958186));
#59698=CARTESIAN_POINT('Ctrl Pts',(13.6259213813758,-21.301925742602,72.0434578858125));
#59699=CARTESIAN_POINT('Ctrl Pts',(13.5472379727687,-20.8952543217083,71.9882997943055));
#59700=CARTESIAN_POINT('Ctrl Pts',(13.4479934727035,-20.6063713493493,71.9205646447771));
#59701=CARTESIAN_POINT('Ctrl Pts',(13.3123339698825,-20.340342487262,71.8314168301733));
#59702=CARTESIAN_POINT('Ctrl Pts',(13.1478804067087,-20.1100991868126,71.7286974247074));
#59703=CARTESIAN_POINT('Ctrl Pts',(12.9619002066534,-19.9164365783173,71.6191149045929));
#59704=CARTESIAN_POINT('Ctrl Pts',(12.7767862629449,-19.7750442233578,71.5174501763976));
#59705=CARTESIAN_POINT('Ctrl Pts',(12.5370551731176,-19.6359411990339,71.3942118174265));
#59706=CARTESIAN_POINT('Ctrl Pts',(12.275131801304,-19.5369293131258,71.2711059537325));
#59707=CARTESIAN_POINT('Ctrl Pts',(11.9573432269876,-19.4882523943241,71.1413575450164));
#59708=CARTESIAN_POINT('Ctrl Pts',(11.6013338289841,-19.4879656798897,71.011543399985));
#59709=CARTESIAN_POINT('Ctrl Pts',(11.1250974427879,-19.5943460899089,70.8696653569674));
#59710=CARTESIAN_POINT('Ctrl Pts',(10.6423938999603,-19.876197434027,70.7673342507931));
#59711=CARTESIAN_POINT('Ctrl Pts',(10.3759502542046,-20.1366682751392,70.7252948452286));
#59712=CARTESIAN_POINT('Ctrl Pts',(10.1892867726256,-20.3739939513888,70.6996355169175));
#59713=CARTESIAN_POINT('Ctrl Pts',(10.0257787789018,-20.637649843183,70.6803473347719));
#59714=CARTESIAN_POINT('Ctrl Pts',(9.8757916185907,-21.0449076219056,70.6663562428006));
#59715=CARTESIAN_POINT('Ctrl Pts',(9.84122986845921,-21.3520059990089,70.6636110875407));
#59716=CARTESIAN_POINT('Ctrl Pts',(9.84122986845921,-21.5,70.6636110875407));
#59717=CARTESIAN_POINT('Ctrl Pts',(9.74287700479826,-21.5,70.5125025877322));
#59718=CARTESIAN_POINT('Ctrl Pts',(9.74287700479826,-21.3437858030339,70.5125025877322));
#59719=CARTESIAN_POINT('Ctrl Pts',(9.77867795084425,-21.0196494588534,70.5144182338898));
#59720=CARTESIAN_POINT('Ctrl Pts',(9.93487527850697,-20.5875814819759,70.5252370307246));
#59721=CARTESIAN_POINT('Ctrl Pts',(10.1066531997307,-20.305521444769,70.5419005952258));
#59722=CARTESIAN_POINT('Ctrl Pts',(10.3040349212154,-20.0501861211832,70.5653346387674));
#59723=CARTESIAN_POINT('Ctrl Pts',(10.5875357806613,-19.7677773346453,70.6053394071194));
#59724=CARTESIAN_POINT('Ctrl Pts',(11.1091117678361,-19.4569229967783,70.7097325311002));
#59725=CARTESIAN_POINT('Ctrl Pts',(11.6310650689274,-19.3376578948939,70.8625951386498));
#59726=CARTESIAN_POINT('Ctrl Pts',(12.0216107241993,-19.338052834614,71.005036372742));
#59727=CARTESIAN_POINT('Ctrl Pts',(12.3693061289729,-19.3924814953289,71.1481752603989));
#59728=CARTESIAN_POINT('Ctrl Pts',(12.6535693601998,-19.5026800844597,71.2842239697829));
#59729=CARTESIAN_POINT('Ctrl Pts',(12.9112681237482,-19.656071853345,71.4199434952884));
#59730=CARTESIAN_POINT('Ctrl Pts',(13.108633737568,-19.8110230421895,71.5315418245281));
#59731=CARTESIAN_POINT('Ctrl Pts',(13.30479452339,-20.0214367560947,71.6512132027746));
#59732=CARTESIAN_POINT('Ctrl Pts',(13.4764722169006,-20.2695559196014,71.7628122981255));
#59733=CARTESIAN_POINT('Ctrl Pts',(13.6166712998014,-20.5540190040535,71.8591758531238));
#59734=CARTESIAN_POINT('Ctrl Pts',(13.7183983186692,-20.8609704899414,71.932093483098));
#59735=CARTESIAN_POINT('Ctrl Pts',(13.7985524061519,-21.2911597238678,71.9912918069344));
#59736=CARTESIAN_POINT('Ctrl Pts',(13.7979233224896,-21.6302708884948,71.9909065809688));
#59737=CARTESIAN_POINT('Ctrl Pts',(13.7535308851104,-21.9512225876456,71.9580350138515));
#59738=CARTESIAN_POINT('Ctrl Pts',(13.709674381118,-22.1641725337909,71.9258725275639));
#59739=CARTESIAN_POINT('Ctrl Pts',(13.6168015105668,-22.4461912796831,71.8592569555153));
#59740=CARTESIAN_POINT('Ctrl Pts',(13.4763850760173,-22.7304324210399,71.7627534820972));
#59741=CARTESIAN_POINT('Ctrl Pts',(13.3051919767247,-22.9780992092235,71.6514654851331));
#59742=CARTESIAN_POINT('Ctrl Pts',(13.1084649034627,-23.1892327479386,71.5314239215564));
#59743=CARTESIAN_POINT('Ctrl Pts',(12.8719512966863,-23.3748625900797,71.3976849620357));
#59744=CARTESIAN_POINT('Ctrl Pts',(12.6510577647346,-23.4940583870137,71.2838949455475));
#59745=CARTESIAN_POINT('Ctrl Pts',(12.4866718330575,-23.5575942766802,71.2055992342487));
#59746=CARTESIAN_POINT('Ctrl Pts',(12.4027779159087,-23.5839664204326,71.167268720936));
#59747=CARTESIAN_POINT('Ctrl Pts',(12.3543904463612,-23.5975235527391,71.1456250307213));
#59748=CARTESIAN_POINT('Ctrl Pts',(12.2208094014591,-23.6319919884316,71.0867018338967));
#59749=CARTESIAN_POINT('Ctrl Pts',(12.0578852179822,-23.6557172786385,71.0201457155622));
#59750=CARTESIAN_POINT('Ctrl Pts',(11.7658252370385,-23.664271882774,70.9111982308898));
#59751=CARTESIAN_POINT('Ctrl Pts',(11.5562073871596,-23.6406588378193,70.8422231900863));
#59752=CARTESIAN_POINT('Ctrl Pts',(11.3646737922248,-23.5926452515457,70.7868530255724));
#59753=CARTESIAN_POINT('Ctrl Pts',(11.2883532161314,-23.5711895983197,70.7654371551999));
#59754=CARTESIAN_POINT('Ctrl Pts',(11.1554284786727,-23.5274756480171,70.7298614280393));
#59755=CARTESIAN_POINT('Ctrl Pts',(10.8954109293732,-23.4174824644433,70.6667169758025));
#59756=CARTESIAN_POINT('Ctrl Pts',(10.5505406389766,-23.1948597886741,70.600128983041));
#59757=CARTESIAN_POINT('Ctrl Pts',(10.2764424102782,-22.9226724124575,70.5614144955755));
#59758=CARTESIAN_POINT('Ctrl Pts',(10.083942330172,-22.6596849246672,70.5396163501376));
#59759=CARTESIAN_POINT('Ctrl Pts',(9.92068473931345,-22.3731848943024,70.5242594183206));
#59760=CARTESIAN_POINT('Ctrl Pts',(9.77861943028971,-21.9803373691276,70.5144059476976));
#59761=CARTESIAN_POINT('Ctrl Pts',(9.74287700479826,-21.656214196966,70.5125025877322));
#59762=CARTESIAN_POINT('Ctrl Pts',(9.74287700479826,-21.5,70.5125025877322));
#59763=CARTESIAN_POINT('Origin',(9.31,-19.775,78.));
#59764=CARTESIAN_POINT('',(1.81,-25.3,78.));
#59765=CARTESIAN_POINT('Origin',(9.31,-25.3,78.));
#59766=CARTESIAN_POINT('',(1.81,-14.25,78.));
#59767=CARTESIAN_POINT('',(1.81,-19.775,78.));
#59768=CARTESIAN_POINT('Origin',(9.31,-14.25,78.));
#59769=CARTESIAN_POINT('',(4.82873245991394,-21.5,84.014003760738));
#59770=CARTESIAN_POINT('Ctrl Pts',(4.82873245991394,-21.5,84.014003760738));
#59771=CARTESIAN_POINT('Ctrl Pts',(4.82873245991394,-21.6562141969661,84.014003760738));
#59772=CARTESIAN_POINT('Ctrl Pts',(4.85736622748711,-21.9803502519472,84.0355447824565));
#59773=CARTESIAN_POINT('Ctrl Pts',(4.98401828163431,-22.4124109055271,84.1276650488678));
#59774=CARTESIAN_POINT('Ctrl Pts',(5.12625478749138,-22.6944732941622,84.2253058354118));
#59775=CARTESIAN_POINT('Ctrl Pts',(5.2926198619563,-22.9497986695551,84.3342442319345));
#59776=CARTESIAN_POINT('Ctrl Pts',(5.53493133383187,-23.2322336732833,84.4857324948551));
#59777=CARTESIAN_POINT('Ctrl Pts',(5.89665156355806,-23.4723187384843,84.6831785101655));
#59778=CARTESIAN_POINT('Ctrl Pts',(6.2753117530903,-23.6086799844817,84.8611083880992));
#59779=CARTESIAN_POINT('Ctrl Pts',(6.57408560510447,-23.662351077972,84.9862512166584));
#59780=CARTESIAN_POINT('Ctrl Pts',(6.89079758792843,-23.6619346851716,85.1014126433423));
#59781=CARTESIAN_POINT('Ctrl Pts',(7.14703055733959,-23.6230346405478,85.1827564818876));
#59782=CARTESIAN_POINT('Ctrl Pts',(7.45300707834779,-23.5382170209426,85.2689305062561));
#59783=CARTESIAN_POINT('Ctrl Pts',(7.75038779391833,-23.4057620043471,85.3390556557566));
#59784=CARTESIAN_POINT('Ctrl Pts',(8.06196599656662,-23.1891502055613,85.3968111581528));
#59785=CARTESIAN_POINT('Ctrl Pts',(8.28948884338796,-22.9784739218892,85.4312988805198));
#59786=CARTESIAN_POINT('Ctrl Pts',(8.47541979746267,-22.7514824404779,85.4540052246341));
#59787=CARTESIAN_POINT('Ctrl Pts',(8.59144124522549,-22.5645860879582,85.4656428345252));
#59788=CARTESIAN_POINT('Ctrl Pts',(8.74391346127118,-22.272332044321,85.4793401936152));
#59789=CARTESIAN_POINT('Ctrl Pts',(8.85381443839301,-21.9240224696184,85.4861466895026));
#59790=CARTESIAN_POINT('Ctrl Pts',(8.87901361505321,-21.5779256266326,85.487614474219));
#59791=CARTESIAN_POINT('Ctrl Pts',(8.87516743536897,-21.3694798611557,85.4873864938745));
#59792=CARTESIAN_POINT('Ctrl Pts',(8.85513326762087,-21.1553648060587,85.48622725368));
#59793=CARTESIAN_POINT('Ctrl Pts',(8.78657759480108,-20.8615791622571,85.4819283317405));
#59794=CARTESIAN_POINT('Ctrl Pts',(8.6617617762221,-20.5533339316959,85.4724237592255));
#59795=CARTESIAN_POINT('Ctrl Pts',(8.53517073786835,-20.3410662633443,85.4602233453799));
#59796=CARTESIAN_POINT('Ctrl Pts',(8.40767692089607,-20.1659139729294,85.4457557150761));
#59797=CARTESIAN_POINT('Ctrl Pts',(8.27089129566994,-20.0045077474062,85.4284509108725));
#59798=CARTESIAN_POINT('Ctrl Pts',(8.06181738257177,-19.8106817132535,85.3968159991057));
#59799=CARTESIAN_POINT('Ctrl Pts',(7.82802168890365,-19.6482675713107,85.3534138355257));
#59800=CARTESIAN_POINT('Ctrl Pts',(7.63726184737735,-19.5478095215932,85.3116066824435));
#59801=CARTESIAN_POINT('Ctrl Pts',(7.48927323429437,-19.4831548365047,85.2760681754352));
#59802=CARTESIAN_POINT('Ctrl Pts',(7.37608465013576,-19.4424658819364,85.2467130241579));
#59803=CARTESIAN_POINT('Ctrl Pts',(7.29030926384011,-19.4169940333725,85.2230170810003));
#59804=CARTESIAN_POINT('Ctrl Pts',(7.25209035941627,-19.406734446681,85.2121572627922));
#59805=CARTESIAN_POINT('Ctrl Pts',(7.2266071958566,-19.4001505834634,85.2048434726207));
#59806=CARTESIAN_POINT('Ctrl Pts',(7.05731504363103,-19.3586067795117,85.1556486945886));
#59807=CARTESIAN_POINT('Ctrl Pts',(6.83602917970007,-19.3336186512925,85.0828499150213));
#59808=CARTESIAN_POINT('Ctrl Pts',(6.54311667666213,-19.3463797210142,84.9723056198425));
#59809=CARTESIAN_POINT('Ctrl Pts',(6.38396293084926,-19.3722629250898,84.9064904925777));
#59810=CARTESIAN_POINT('Ctrl Pts',(6.27463875524686,-19.4001766884773,84.8583531527386));
#59811=CARTESIAN_POINT('Ctrl Pts',(6.2428188528774,-19.4088188503593,84.8441968000193));
#59812=CARTESIAN_POINT('Ctrl Pts',(6.21570312034965,-19.4167674428179,84.8319688066155));
#59813=CARTESIAN_POINT('Ctrl Pts',(6.16169834482935,-19.4335244855137,84.807359990206));
#59814=CARTESIAN_POINT('Ctrl Pts',(6.05042792170448,-19.472436531396,84.7554486067052));
#59815=CARTESIAN_POINT('Ctrl Pts',(5.84476190630921,-19.5673683139041,84.653489704449));
#59816=CARTESIAN_POINT('Ctrl Pts',(5.65739800951548,-19.6930263775506,84.5515530734112));
#59817=CARTESIAN_POINT('Ctrl Pts',(5.43315068978185,-19.8873972581003,84.4219190497216));
#59818=CARTESIAN_POINT('Ctrl Pts',(5.26897645452575,-20.0769606002621,84.319589452044));
#59819=CARTESIAN_POINT('Ctrl Pts',(5.10741908303976,-20.3403380172447,84.2124573333873));
#59820=CARTESIAN_POINT('Ctrl Pts',(4.97251341135122,-20.6267209881876,84.1193109715028));
#59821=CARTESIAN_POINT('Ctrl Pts',(4.85732795150402,-21.0196848429533,84.0355138144579));
#59822=CARTESIAN_POINT('Ctrl Pts',(4.82873245991394,-21.3437858030339,84.014003760738));
#59823=CARTESIAN_POINT('Ctrl Pts',(4.82873245991394,-21.5,84.014003760738));
#59824=CARTESIAN_POINT('',(16.6267263258151,-16.3,79.6478822388519));
#59825=CARTESIAN_POINT('Ctrl Pts',(16.6267263258151,-16.3,79.6478822388519));
#59826=CARTESIAN_POINT('Ctrl Pts',(16.6267263258151,-16.1627202519724,79.6478822388519));
#59827=CARTESIAN_POINT('Ctrl Pts',(16.6179955133542,-15.9782014756465,79.6876782461328));
#59828=CARTESIAN_POINT('Ctrl Pts',(16.5950312459286,-15.8037451346603,79.7828728219127));
#59829=CARTESIAN_POINT('Ctrl Pts',(16.586544255709,-15.7515481629588,79.8170540818662));
#59830=CARTESIAN_POINT('Ctrl Pts',(16.5813766158318,-15.7228477592171,79.837607390227));
#59831=CARTESIAN_POINT('Ctrl Pts',(16.5678845354643,-15.6528601133616,79.8907518590427));
#59832=CARTESIAN_POINT('Ctrl Pts',(16.548100587601,-15.5753837738119,79.9659216531079));
#59833=CARTESIAN_POINT('Ctrl Pts',(16.5162719674538,-15.4912042488478,80.0789622080761));
#59834=CARTESIAN_POINT('Ctrl Pts',(16.4893053796703,-15.438486627179,80.1703295926858));
#59835=CARTESIAN_POINT('Ctrl Pts',(16.4643631140139,-15.4034928690422,80.2509476732841));
#59836=CARTESIAN_POINT('Ctrl Pts',(16.4458365951828,-15.3843016285567,80.3086730273532));
#59837=CARTESIAN_POINT('Ctrl Pts',(16.4363274974597,-15.3760122112162,80.3377790265208));
#59838=CARTESIAN_POINT('Ctrl Pts',(16.4308398851589,-15.371663215768,80.3544280421398));
#59839=CARTESIAN_POINT('Ctrl Pts',(16.4058754210574,-15.353224391122,80.4297068102671));
#59840=CARTESIAN_POINT('Ctrl Pts',(16.3586107169648,-15.3376504708956,80.5654454852136));
#59841=CARTESIAN_POINT('Ctrl Pts',(16.308363242307,-15.3529640814669,80.6977276874573));
#59842=CARTESIAN_POINT('Ctrl Pts',(16.2807580438145,-15.37010041347,80.7673524199429));
#59843=CARTESIAN_POINT('Ctrl Pts',(16.2775147617408,-15.3721798545712,80.7755097810832));
#59844=CARTESIAN_POINT('Ctrl Pts',(16.2734481412606,-15.3748990742495,80.7856999038481));
#59845=CARTESIAN_POINT('Ctrl Pts',(16.2685609643578,-15.3783529418162,80.7978834589029));
#59846=CARTESIAN_POINT('Ctrl Pts',(16.2620326141532,-15.3832121080572,80.8140766685934));
#59847=CARTESIAN_POINT('Ctrl Pts',(16.2554916800538,-15.388450767397,80.8301796061662));
#59848=CARTESIAN_POINT('Ctrl Pts',(16.248947338163,-15.3940656126707,80.8461713540943));
#59849=CARTESIAN_POINT('Ctrl Pts',(16.2325860018634,-15.4087182634758,80.8859576775251));
#59850=CARTESIAN_POINT('Ctrl Pts',(16.2047961808524,-15.4384721428059,80.952041722185));
#59851=CARTESIAN_POINT('Ctrl Pts',(16.1666865284266,-15.4912543308356,81.0394472234925));
#59852=CARTESIAN_POINT('Ctrl Pts',(16.1185975434662,-15.5751968380705,81.1460824099368));
#59853=CARTESIAN_POINT('Ctrl Pts',(16.0669428124562,-15.6953850753735,81.2556190750553));
#59854=CARTESIAN_POINT('Ctrl Pts',(16.0200372266792,-15.8604273231654,81.3507157648354));
#59855=CARTESIAN_POINT('Ctrl Pts',(15.9959680144551,-15.996365623908,81.3982024054527));
#59856=CARTESIAN_POINT('Ctrl Pts',(15.9859992260481,-16.0782746472634,81.4177123723923));
#59857=CARTESIAN_POINT('Ctrl Pts',(15.981559283011,-16.1252411321897,81.4263653146201));
#59858=CARTESIAN_POINT('Ctrl Pts',(15.9725425009045,-16.2435059768007,81.4438943965471));
#59859=CARTESIAN_POINT('Ctrl Pts',(15.9726062552113,-16.3565449674897,81.443748920257));
#59860=CARTESIAN_POINT('Ctrl Pts',(15.9816103595508,-16.4745965934211,81.4262469365913));
#59861=CARTESIAN_POINT('Ctrl Pts',(15.9860578245946,-16.5216040414588,81.4175766075504));
#59862=CARTESIAN_POINT('Ctrl Pts',(15.9931529411453,-16.5800659147356,81.4036970257625));
#59863=CARTESIAN_POINT('Ctrl Pts',(16.0022521358187,-16.6373793785181,81.3857696123251));
#59864=CARTESIAN_POINT('Ctrl Pts',(16.0106538593799,-16.6821981103206,81.3691011936988));
#59865=CARTESIAN_POINT('Ctrl Pts',(16.0334936810962,-16.7925239444982,81.3235736952026));
#59866=CARTESIAN_POINT('Ctrl Pts',(16.0732729417727,-16.9216470840919,81.2426097135714));
#59867=CARTESIAN_POINT('Ctrl Pts',(16.1302272700693,-17.0466007917327,81.1205411519808));
#59868=CARTESIAN_POINT('Ctrl Pts',(16.1791754703243,-17.1289822618776,81.0115059847778));
#59869=CARTESIAN_POINT('Ctrl Pts',(16.2223085872669,-17.1816622921672,80.9108472236554));
#59870=CARTESIAN_POINT('Ctrl Pts',(16.2529286652786,-17.2096866928451,80.8365863008715));
#59871=CARTESIAN_POINT('Ctrl Pts',(16.2703393347549,-17.2229799642533,80.7935103025339));
#59872=CARTESIAN_POINT('Ctrl Pts',(16.3311939963963,-17.263076777122,80.640871035239));
#59873=CARTESIAN_POINT('Ctrl Pts',(16.3879482597749,-17.2633110844262,80.4849293868592));
#59874=CARTESIAN_POINT('Ctrl Pts',(16.4430881666924,-17.2186801784522,80.3172431103551));
#59875=CARTESIAN_POINT('Ctrl Pts',(16.4642217393025,-17.1966318363056,80.251361487145));
#59876=CARTESIAN_POINT('Ctrl Pts',(16.4991469954625,-17.1481299251104,80.1385791791468));
#59877=CARTESIAN_POINT('Ctrl Pts',(16.5417979890631,-17.0491114348861,79.9898247024023));
#59878=CARTESIAN_POINT('Ctrl Pts',(16.5787193153288,-16.9047265894586,79.8495489824192));
#59879=CARTESIAN_POINT('Ctrl Pts',(16.6070569699324,-16.7195440420054,79.7337450825527));
#59880=CARTESIAN_POINT('Ctrl Pts',(16.6232895344097,-16.5114662207145,79.6631181782204));
#59881=CARTESIAN_POINT('Ctrl Pts',(16.6267263258151,-16.3686398740138,79.647882238852));
#59882=CARTESIAN_POINT('Ctrl Pts',(16.6267263258151,-16.3,79.647882238852));
#59883=CARTESIAN_POINT('Origin',(9.31513030214989,-21.5,77.9859046106882));
#59884=CARTESIAN_POINT('',(5.00120579598144,-21.5,83.9614679362901));
#59885=CARTESIAN_POINT('',(7.42634813437021,-21.5,77.2984441226036));
#59886=CARTESIAN_POINT('Ctrl Pts',(5.00120579598144,-21.5,83.9614679362901));
#59887=CARTESIAN_POINT('Ctrl Pts',(5.00120579598144,-21.3520059990089,83.9614679362901));
#59888=CARTESIAN_POINT('Ctrl Pts',(5.02938710354273,-21.0449379529334,83.9815481249973));
#59889=CARTESIAN_POINT('Ctrl Pts',(5.14210001521926,-20.6745440882475,84.0595031650574));
#59890=CARTESIAN_POINT('Ctrl Pts',(5.27274890176333,-20.4064934480325,84.1457116731447));
#59891=CARTESIAN_POINT('Ctrl Pts',(5.42805833516398,-20.1613379356766,84.2445019203697));
#59892=CARTESIAN_POINT('Ctrl Pts',(5.5842076611768,-19.9865699045241,84.3383374923964));
#59893=CARTESIAN_POINT('Ctrl Pts',(5.79518871998536,-19.8086662168602,84.4566186593402));
#59894=CARTESIAN_POINT('Ctrl Pts',(5.97008028592641,-19.6944825986058,84.5492829143672));
#59895=CARTESIAN_POINT('Ctrl Pts',(6.16024874649474,-19.6088242840925,84.6416704339889));
#59896=CARTESIAN_POINT('Ctrl Pts',(6.26265561097925,-19.5738308190456,84.6886756114093));
#59897=CARTESIAN_POINT('Ctrl Pts',(6.31228285326648,-19.5587773020503,84.7109583986528));
#59898=CARTESIAN_POINT('Ctrl Pts',(6.33718439395397,-19.5516405475664,84.7220307194513));
#59899=CARTESIAN_POINT('Ctrl Pts',(6.36638310919858,-19.5438854025941,84.7348502432122));
#59900=CARTESIAN_POINT('Ctrl Pts',(6.46664380786896,-19.5188490700099,84.7784451622438));
#59901=CARTESIAN_POINT('Ctrl Pts',(6.61214355835411,-19.4956974788605,84.8381010128625));
#59902=CARTESIAN_POINT('Ctrl Pts',(6.87934184713117,-19.4843021730789,84.9386886521805));
#59903=CARTESIAN_POINT('Ctrl Pts',(7.08098376058415,-19.5065990278365,85.0055173198125));
#59904=CARTESIAN_POINT('Ctrl Pts',(7.23572536065315,-19.5438603297829,85.0512669854069));
#59905=CARTESIAN_POINT('Ctrl Pts',(7.25902594561429,-19.5497685575946,85.0580779380141));
#59906=CARTESIAN_POINT('Ctrl Pts',(7.29398062082609,-19.5589776728157,85.068202640782));
#59907=CARTESIAN_POINT('Ctrl Pts',(7.37249143930395,-19.5818620333112,85.0903671757502));
#59908=CARTESIAN_POINT('Ctrl Pts',(7.47629543310783,-19.6184900161799,85.1180421488052));
#59909=CARTESIAN_POINT('Ctrl Pts',(7.61240028365782,-19.6768804536723,85.1519024555482));
#59910=CARTESIAN_POINT('Ctrl Pts',(7.7884588882969,-19.7679209606644,85.1922855511176));
#59911=CARTESIAN_POINT('Ctrl Pts',(8.00571902094384,-19.9161198082099,85.2354092037281));
#59912=CARTESIAN_POINT('Ctrl Pts',(8.20165416446568,-20.0945202553182,85.2681402867983));
#59913=CARTESIAN_POINT('Ctrl Pts',(8.33072651652134,-20.2441651242008,85.2867918154456));
#59914=CARTESIAN_POINT('Ctrl Pts',(8.45148795656648,-20.4072154069382,85.3028209480783));
#59915=CARTESIAN_POINT('Ctrl Pts',(8.57200758743931,-20.6057239697199,85.3169691524854));
#59916=CARTESIAN_POINT('Ctrl Pts',(8.69159825227611,-20.8958285905613,85.3288534467772));
#59917=CARTESIAN_POINT('Ctrl Pts',(8.75757356805284,-21.1735479434414,85.3346262878536));
#59918=CARTESIAN_POINT('Ctrl Pts',(8.77688460061852,-21.3763469753939,85.336233820364));
#59919=CARTESIAN_POINT('Ctrl Pts',(8.78059087654672,-21.5738186910076,85.3365468413902));
#59920=CARTESIAN_POINT('Ctrl Pts',(8.75630061671194,-21.9017339681359,85.334517176155));
#59921=CARTESIAN_POINT('Ctrl Pts',(8.65051985500575,-22.2305671395078,85.3253318026369));
#59922=CARTESIAN_POINT('Ctrl Pts',(8.50506066967912,-22.5045527127309,85.3091069381655));
#59923=CARTESIAN_POINT('Ctrl Pts',(8.39473328732379,-22.6791889660986,85.2957679284494));
#59924=CARTESIAN_POINT('Ctrl Pts',(8.21907518119456,-22.8898206522999,85.2710792257392));
#59925=CARTESIAN_POINT('Ctrl Pts',(8.00586508617554,-23.0837282560587,85.2354108414265));
#59926=CARTESIAN_POINT('Ctrl Pts',(7.71630377271468,-23.2813748438679,85.1780083266107));
#59927=CARTESIAN_POINT('Ctrl Pts',(7.44278857103648,-23.4008177940264,85.1110366251592));
#59928=CARTESIAN_POINT('Ctrl Pts',(7.16292149566871,-23.476956232333,85.0306247350017));
#59929=CARTESIAN_POINT('Ctrl Pts',(6.92920042935146,-23.5117274127833,84.9556727639564));
#59930=CARTESIAN_POINT('Ctrl Pts',(6.64052521451068,-23.5121075528597,84.8507009698725));
#59931=CARTESIAN_POINT('Ctrl Pts',(6.36728513118301,-23.4641122791779,84.7373259615023));
#59932=CARTESIAN_POINT('Ctrl Pts',(6.01870899323939,-23.3415395005,84.5762647242888));
#59933=CARTESIAN_POINT('Ctrl Pts',(5.68113207878283,-23.1237730049189,84.396893955329));
#59934=CARTESIAN_POINT('Ctrl Pts',(5.45052492150888,-22.8633215721594,84.2579345062791));
#59935=CARTESIAN_POINT('Ctrl Pts',(5.29094963212753,-22.6259977123551,84.1575892563859));
#59936=CARTESIAN_POINT('Ctrl Pts',(5.15335516091919,-22.362344512459,84.0672755210376));
#59937=CARTESIAN_POINT('Ctrl Pts',(5.02942559621785,-21.9550903286244,83.9815767221747));
#59938=CARTESIAN_POINT('Ctrl Pts',(5.00120579598144,-21.6479940009911,83.9614679362901));
#59939=CARTESIAN_POINT('Ctrl Pts',(5.00120579598144,-21.5,83.9614679362901));
#59940=CARTESIAN_POINT('',(8.46456668098594,-23.4399831912377,78.7854630291158));
#59941=CARTESIAN_POINT('',(9.16725530571964,-23.439990633261,76.8549480800671));
#59942=CARTESIAN_POINT('',(8.82100921955859,-23.44,77.8060592445016));
#59943=CARTESIAN_POINT('',(10.1553645548646,-23.43992588449,77.2145815988743));
#59944=CARTESIAN_POINT('Ctrl Pts',(10.1553531683805,-23.4399183977911,77.2145896236657));
#59945=CARTESIAN_POINT('Ctrl Pts',(10.0879810015635,-23.4637967282797,77.1412715498725));
#59946=CARTESIAN_POINT('Ctrl Pts',(9.9717328772446,-23.4927472120551,77.0438930991871));
#59947=CARTESIAN_POINT('Ctrl Pts',(9.76844966013923,-23.5119591404095,76.9341462709327));
#59948=CARTESIAN_POINT('Ctrl Pts',(9.58984999260555,-23.5101434522743,76.872532168987));
#59949=CARTESIAN_POINT('Ctrl Pts',(9.3788902833647,-23.4855876966743,76.8415124408269));
#59950=CARTESIAN_POINT('Ctrl Pts',(9.2427353924026,-23.4580865891214,76.8456230088964));
#59951=CARTESIAN_POINT('Ctrl Pts',(9.17328487982263,-23.4414541894188,76.854157385364));
#59952=CARTESIAN_POINT('Ctrl Pts',(9.16725530571964,-23.439990633261,76.8549480800671));
#59953=CARTESIAN_POINT('',(9.45274488900745,-23.4399725752062,79.1450870611007));
#59954=CARTESIAN_POINT('',(9.80925138474118,-23.44,78.1657499768748));
#59955=CARTESIAN_POINT('Ctrl Pts',(8.46456668098594,-23.4399831912377,78.7854630291158));
#59956=CARTESIAN_POINT('Ctrl Pts',(8.48862373486699,-23.4485471463589,78.8117034392736));
#59957=CARTESIAN_POINT('Ctrl Pts',(8.55980178672779,-23.4709295638718,78.8823074031271));
#59958=CARTESIAN_POINT('Ctrl Pts',(8.69364486134355,-23.4983842652002,78.9832904164185));
#59959=CARTESIAN_POINT('Ctrl Pts',(8.86630044007771,-23.5123967187664,79.0720196330274));
#59960=CARTESIAN_POINT('Ctrl Pts',(9.04620851329942,-23.5082837204292,79.1299209668847));
#59961=CARTESIAN_POINT('Ctrl Pts',(9.24114419357868,-23.4856018928221,79.1585650126785));
#59962=CARTESIAN_POINT('Ctrl Pts',(9.3772214843187,-23.4580769550451,79.1543912360021));
#59963=CARTESIAN_POINT('Ctrl Pts',(9.44668059476406,-23.4414315376984,79.1458387644055));
#59964=CARTESIAN_POINT('Ctrl Pts',(9.45273622862353,-23.4399606993813,79.1450431018916));
#59965=CARTESIAN_POINT('Ctrl Pts',(4.82873245991394,-21.5,84.014003760738));
#59966=CARTESIAN_POINT('Ctrl Pts',(4.82873245991394,-21.3437858030339,84.014003760738));
#59967=CARTESIAN_POINT('Ctrl Pts',(4.85732795150402,-21.0196848429533,84.0355138144579));
#59968=CARTESIAN_POINT('Ctrl Pts',(4.97251341135122,-20.6267209881876,84.1193109715028));
#59969=CARTESIAN_POINT('Ctrl Pts',(5.10741908303976,-20.3403380172447,84.2124573333873));
#59970=CARTESIAN_POINT('Ctrl Pts',(5.26897645452575,-20.0769606002621,84.319589452044));
#59971=CARTESIAN_POINT('Ctrl Pts',(5.43315068978185,-19.8873972581003,84.4219190497216));
#59972=CARTESIAN_POINT('Ctrl Pts',(5.65739800951548,-19.6930263775506,84.5515530734112));
#59973=CARTESIAN_POINT('Ctrl Pts',(5.84476190630921,-19.5673683139041,84.653489704449));
#59974=CARTESIAN_POINT('Ctrl Pts',(6.05042792170448,-19.472436531396,84.7554486067052));
#59975=CARTESIAN_POINT('Ctrl Pts',(6.16169834482935,-19.4335244855137,84.807359990206));
#59976=CARTESIAN_POINT('Ctrl Pts',(6.21570312034965,-19.4167674428179,84.8319688066155));
#59977=CARTESIAN_POINT('Ctrl Pts',(6.2428188528774,-19.4088188503593,84.8441968000193));
#59978=CARTESIAN_POINT('Ctrl Pts',(6.27463875524686,-19.4001766884773,84.8583531527386));
#59979=CARTESIAN_POINT('Ctrl Pts',(6.38396293084926,-19.3722629250898,84.9064904925777));
#59980=CARTESIAN_POINT('Ctrl Pts',(6.54311667666213,-19.3463797210142,84.9723056198425));
#59981=CARTESIAN_POINT('Ctrl Pts',(6.83602917970007,-19.3336186512925,85.0828499150213));
#59982=CARTESIAN_POINT('Ctrl Pts',(7.05731504363103,-19.3586067795117,85.1556486945886));
#59983=CARTESIAN_POINT('Ctrl Pts',(7.2266071958566,-19.4001505834634,85.2048434726207));
#59984=CARTESIAN_POINT('Ctrl Pts',(7.25209035941627,-19.406734446681,85.2121572627922));
#59985=CARTESIAN_POINT('Ctrl Pts',(7.29030926384011,-19.4169940333725,85.2230170810003));
#59986=CARTESIAN_POINT('Ctrl Pts',(7.37608465013576,-19.4424658819364,85.2467130241579));
#59987=CARTESIAN_POINT('Ctrl Pts',(7.48927323429437,-19.4831548365047,85.2760681754352));
#59988=CARTESIAN_POINT('Ctrl Pts',(7.63726184737735,-19.5478095215932,85.3116066824435));
#59989=CARTESIAN_POINT('Ctrl Pts',(7.82802168890365,-19.6482675713107,85.3534138355257));
#59990=CARTESIAN_POINT('Ctrl Pts',(8.06181738257177,-19.8106817132535,85.3968159991057));
#59991=CARTESIAN_POINT('Ctrl Pts',(8.27089129566994,-20.0045077474062,85.4284509108725));
#59992=CARTESIAN_POINT('Ctrl Pts',(8.40767692089607,-20.1659139729294,85.4457557150761));
#59993=CARTESIAN_POINT('Ctrl Pts',(8.53517073786835,-20.3410662633443,85.4602233453799));
#59994=CARTESIAN_POINT('Ctrl Pts',(8.6617617762221,-20.5533339316959,85.4724237592255));
#59995=CARTESIAN_POINT('Ctrl Pts',(8.78657759480108,-20.8615791622571,85.4819283317405));
#59996=CARTESIAN_POINT('Ctrl Pts',(8.85513326762087,-21.1553648060587,85.48622725368));
#59997=CARTESIAN_POINT('Ctrl Pts',(8.87516743536897,-21.3694798611557,85.4873864938745));
#59998=CARTESIAN_POINT('Ctrl Pts',(8.87901361505321,-21.5779256266326,85.487614474219));
#59999=CARTESIAN_POINT('Ctrl Pts',(8.85381443839301,-21.9240224696184,85.4861466895026));
#60000=CARTESIAN_POINT('Ctrl Pts',(8.74391346127118,-22.272332044321,85.4793401936152));
#60001=CARTESIAN_POINT('Ctrl Pts',(8.59144124522549,-22.5645860879582,85.4656428345252));
#60002=CARTESIAN_POINT('Ctrl Pts',(8.47541979746267,-22.7514824404779,85.4540052246341));
#60003=CARTESIAN_POINT('Ctrl Pts',(8.28948884338796,-22.9784739218892,85.4312988805198));
#60004=CARTESIAN_POINT('Ctrl Pts',(8.06196599656662,-23.1891502055613,85.3968111581528));
#60005=CARTESIAN_POINT('Ctrl Pts',(7.75038779391833,-23.4057620043471,85.3390556557566));
#60006=CARTESIAN_POINT('Ctrl Pts',(7.45300707834779,-23.5382170209426,85.2689305062561));
#60007=CARTESIAN_POINT('Ctrl Pts',(7.14703055733959,-23.6230346405478,85.1827564818876));
#60008=CARTESIAN_POINT('Ctrl Pts',(6.89079758792843,-23.6619346851716,85.1014126433423));
#60009=CARTESIAN_POINT('Ctrl Pts',(6.57408560510447,-23.662351077972,84.9862512166584));
#60010=CARTESIAN_POINT('Ctrl Pts',(6.2753117530903,-23.6086799844817,84.8611083880992));
#60011=CARTESIAN_POINT('Ctrl Pts',(5.89665156355806,-23.4723187384843,84.6831785101655));
#60012=CARTESIAN_POINT('Ctrl Pts',(5.53493133383187,-23.2322336732833,84.4857324948551));
#60013=CARTESIAN_POINT('Ctrl Pts',(5.2926198619563,-22.9497986695551,84.3342442319345));
#60014=CARTESIAN_POINT('Ctrl Pts',(5.12625478749138,-22.6944732941622,84.2253058354118));
#60015=CARTESIAN_POINT('Ctrl Pts',(4.98401828163431,-22.4124109055271,84.1276650488678));
#60016=CARTESIAN_POINT('Ctrl Pts',(4.85736622748711,-21.9803502519472,84.0355447824565));
#60017=CARTESIAN_POINT('Ctrl Pts',(4.82873245991394,-21.6562141969661,84.014003760738));
#60018=CARTESIAN_POINT('Ctrl Pts',(4.82873245991394,-21.5,84.014003760738));
#60019=CARTESIAN_POINT('Ctrl Pts',(4.88622357193644,-21.5,83.9964918192554));
#60020=CARTESIAN_POINT('Ctrl Pts',(4.88622357193644,-21.3465258683589,83.9964918192554));
#60021=CARTESIAN_POINT('Ctrl Pts',(4.91468100218359,-21.02810254628,84.0175252513044));
#60022=CARTESIAN_POINT('Ctrl Pts',(5.02904227930723,-20.6426620215409,84.099375036021));
#60023=CARTESIAN_POINT('Ctrl Pts',(5.16252902261428,-20.3623898275073,84.1902087799731));
#60024=CARTESIAN_POINT('Ctrl Pts',(5.32200374807183,-20.1050863787336,84.2945602748192));
#60025=CARTESIAN_POINT('Ctrl Pts',(5.48350301358017,-19.9204548069083,84.3940585306133));
#60026=CARTESIAN_POINT('Ctrl Pts',(5.70332824633877,-19.7315729906538,84.5199082687209));
#60027=CARTESIAN_POINT('Ctrl Pts',(5.88653469951494,-19.609739742138,84.6187541077551));
#60028=CARTESIAN_POINT('Ctrl Pts',(6.08703486330123,-19.5178991156282,84.7175225491331));
#60029=CARTESIAN_POINT('Ctrl Pts',(6.19535076687932,-19.4802932633577,84.7677985306071));
#60030=CARTESIAN_POINT('Ctrl Pts',(6.24789636465526,-19.464104062562,84.7916320039613));
#60031=CARTESIAN_POINT('Ctrl Pts',(6.27427403323625,-19.4564260827617,84.8034747731633));
#60032=CARTESIAN_POINT('Ctrl Pts',(6.3052202065641,-19.4480795931829,84.8171855162298));
#60033=CARTESIAN_POINT('Ctrl Pts',(6.41152322318916,-19.4211249733965,84.8638087157997));
#60034=CARTESIAN_POINT('Ctrl Pts',(6.56612563722612,-19.396152306963,84.9275707508492));
#60035=CARTESIAN_POINT('Ctrl Pts',(6.85046673551044,-19.383846491888,85.034796160741));
#60036=CARTESIAN_POINT('Ctrl Pts',(7.06520461594874,-19.4079375289533,85.1056049029966));
#60037=CARTESIAN_POINT('Ctrl Pts',(7.22964658412212,-19.4480538322366,85.1536513102161));
#60038=CARTESIAN_POINT('Ctrl Pts',(7.25440222148228,-19.4544124836522,85.1607974878662));
#60039=CARTESIAN_POINT('Ctrl Pts',(7.29153304950211,-19.4643219131869,85.1714122675942));
#60040=CARTESIAN_POINT('Ctrl Pts',(7.37488691319182,-19.488931265728,85.1945977413554));
#60041=CARTESIAN_POINT('Ctrl Pts',(7.48494730056552,-19.5282665630631,85.2233928332252));
#60042=CARTESIAN_POINT('Ctrl Pts',(7.62897465947084,-19.5908331656196,85.258371940145));
#60043=CARTESIAN_POINT('Ctrl Pts',(7.8148340887014,-19.6881520344286,85.2997044073897));
#60044=CARTESIAN_POINT('Ctrl Pts',(8.04311792869579,-19.8458277449056,85.3430137339799));
#60045=CARTESIAN_POINT('Ctrl Pts',(8.24781225193518,-20.0345119167102,85.3750140361811));
#60046=CARTESIAN_POINT('Ctrl Pts',(8.38202678610449,-20.1919976900199,85.3927677485326));
#60047=CARTESIAN_POINT('Ctrl Pts',(8.50727647743439,-20.3631159778756,85.4077558796127));
#60048=CARTESIAN_POINT('Ctrl Pts',(8.6318437132945,-20.5707972777039,85.4206055569788));
#60049=CARTESIAN_POINT('Ctrl Pts',(8.75491781395942,-20.8729956383585,85.4309033700861));
#60050=CARTESIAN_POINT('Ctrl Pts',(8.82261336776486,-21.161425851853,85.4356935984045));
#60051=CARTESIAN_POINT('Ctrl Pts',(8.84240649045215,-21.3717688992351,85.437002269371));
#60052=CARTESIAN_POINT('Ctrl Pts',(8.84620603555104,-21.5765566480909,85.4372585966094));
#60053=CARTESIAN_POINT('Ctrl Pts',(8.82130983116599,-21.9165929691243,85.4356035183868));
#60054=CARTESIAN_POINT('Ctrl Pts',(8.7127822591827,-22.2584104093833,85.4280040632891));
#60055=CARTESIAN_POINT('Ctrl Pts',(8.56264772004336,-22.5445749628824,85.4134642024053));
#60056=CARTESIAN_POINT('Ctrl Pts',(8.44852429408304,-22.7273846156848,85.4012594592392));
#60057=CARTESIAN_POINT('Ctrl Pts',(8.26601762265683,-22.9489228320261,85.3778923289262));
#60058=CARTESIAN_POINT('Ctrl Pts',(8.04326569310293,-23.1540095557271,85.3430110525773));
#60059=CARTESIAN_POINT('Ctrl Pts',(7.73902645351712,-23.3642996175207,85.285373212708));
#60060=CARTESIAN_POINT('Ctrl Pts',(7.44960090924402,-23.4924172786372,85.2162992125571));
#60061=CARTESIAN_POINT('Ctrl Pts',(7.15232753678263,-23.5743418378095,85.1320458995923));
#60062=CARTESIAN_POINT('Ctrl Pts',(6.90359853506944,-23.6118655943755,85.052832683547));
#60063=CARTESIAN_POINT('Ctrl Pts',(6.59623214157321,-23.6122699029346,84.9410678010631));
#60064=CARTESIAN_POINT('Ctrl Pts',(6.30596954578787,-23.5604907493805,84.8198475792336));
#60065=CARTESIAN_POINT('Ctrl Pts',(5.93733737345184,-23.4287256591562,84.6475405815399));
#60066=CARTESIAN_POINT('Ctrl Pts',(5.58366491548219,-23.1960801171618,84.4561196483464));
#60067=CARTESIAN_POINT('Ctrl Pts',(5.34525488180716,-22.9209729704232,84.308807656716));
#60068=CARTESIAN_POINT('Ctrl Pts',(5.18115306903677,-22.6716481002265,84.2027336424032));
#60069=CARTESIAN_POINT('Ctrl Pts',(5.0404639080626,-22.3957221078377,84.1075352062577));
#60070=CARTESIAN_POINT('Ctrl Pts',(4.91471935039736,-21.9719302775063,84.0175554290292));
#60071=CARTESIAN_POINT('Ctrl Pts',(4.88622357193644,-21.6534741316411,83.9964918192554));
#60072=CARTESIAN_POINT('Ctrl Pts',(4.88622357193644,-21.5,83.9964918192554));
#60073=CARTESIAN_POINT('Ctrl Pts',(4.94371468395894,-21.5,83.9789798777728));
#60074=CARTESIAN_POINT('Ctrl Pts',(4.94371468395894,-21.3492659336839,83.9789798777728));
#60075=CARTESIAN_POINT('Ctrl Pts',(4.97203405286316,-21.0365202496067,83.9995366881508));
#60076=CARTESIAN_POINT('Ctrl Pts',(5.08557114726325,-20.6586030548942,84.0794391005392));
#60077=CARTESIAN_POINT('Ctrl Pts',(5.2176389621888,-20.3844416377699,84.1679602265589));
#60078=CARTESIAN_POINT('Ctrl Pts',(5.3750310416179,-20.1332121572051,84.2695310975945));
#60079=CARTESIAN_POINT('Ctrl Pts',(5.53385533737848,-19.9535123557162,84.3661980115048));
#60080=CARTESIAN_POINT('Ctrl Pts',(5.74925848316206,-19.770119603757,84.4882634640305));
#60081=CARTESIAN_POINT('Ctrl Pts',(5.92830749272068,-19.6521111703719,84.5840185110611));
#60082=CARTESIAN_POINT('Ctrl Pts',(6.12364180489798,-19.5633616998603,84.6795964915611));
#60083=CARTESIAN_POINT('Ctrl Pts',(6.22900318892928,-19.5270620412017,84.7282370710082));
#60084=CARTESIAN_POINT('Ctrl Pts',(6.28008960896087,-19.5114406823062,84.7512952013071));
#60085=CARTESIAN_POINT('Ctrl Pts',(6.30572921359511,-19.5040333151641,84.7627527463073));
#60086=CARTESIAN_POINT('Ctrl Pts',(6.33580165788134,-19.4959824978885,84.776017879721));
#60087=CARTESIAN_POINT('Ctrl Pts',(6.43908351552906,-19.4699870217032,84.8211269390218));
#60088=CARTESIAN_POINT('Ctrl Pts',(6.58913459779012,-19.4459248929117,84.8828358818558));
#60089=CARTESIAN_POINT('Ctrl Pts',(6.8649042913208,-19.4340743324834,84.9867424064607));
#60090=CARTESIAN_POINT('Ctrl Pts',(7.07309418826644,-19.4572682783949,85.0555611114046));
#60091=CARTESIAN_POINT('Ctrl Pts',(7.23268597238763,-19.4959570810097,85.1024591478115));
#60092=CARTESIAN_POINT('Ctrl Pts',(7.25671408354828,-19.5020905206234,85.1094377129401));
#60093=CARTESIAN_POINT('Ctrl Pts',(7.2927568351641,-19.5116497930013,85.1198074541881));
#60094=CARTESIAN_POINT('Ctrl Pts',(7.37368917624788,-19.5353966495196,85.1424824585528));
#60095=CARTESIAN_POINT('Ctrl Pts',(7.48062136683667,-19.5733782896215,85.1707174910152));
#60096=CARTESIAN_POINT('Ctrl Pts',(7.62068747156432,-19.6338568096459,85.2051371978466));
#60097=CARTESIAN_POINT('Ctrl Pts',(7.80164648849915,-19.7280364975465,85.2459949792536));
#60098=CARTESIAN_POINT('Ctrl Pts',(8.02441847481981,-19.8809737765578,85.289211468854));
#60099=CARTESIAN_POINT('Ctrl Pts',(8.22473320820043,-20.0645160860142,85.3215771614897));
#60100=CARTESIAN_POINT('Ctrl Pts',(8.35637665131292,-20.2180814071103,85.3397797819891));
#60101=CARTESIAN_POINT('Ctrl Pts',(8.47938221700044,-20.3851656924069,85.3552884138455));
#60102=CARTESIAN_POINT('Ctrl Pts',(8.60192565036691,-20.5882606237119,85.3687873547321));
#60103=CARTESIAN_POINT('Ctrl Pts',(8.72325803311777,-20.8844121144599,85.3798784084316));
#60104=CARTESIAN_POINT('Ctrl Pts',(8.79009346790885,-21.1674868976472,85.385159943129));
#60105=CARTESIAN_POINT('Ctrl Pts',(8.80964554553534,-21.3740579373145,85.3866180448675));
#60106=CARTESIAN_POINT('Ctrl Pts',(8.81339845604888,-21.5751876695492,85.3869027189998));
#60107=CARTESIAN_POINT('Ctrl Pts',(8.78880522393897,-21.9091634686301,85.3850603472709));
#60108=CARTESIAN_POINT('Ctrl Pts',(8.68165105709423,-22.2444887744455,85.376667932963));
#60109=CARTESIAN_POINT('Ctrl Pts',(8.53385419486124,-22.5245638378067,85.3612855702854));
#60110=CARTESIAN_POINT('Ctrl Pts',(8.42162879070342,-22.7032867908917,85.3485136938443));
#60111=CARTESIAN_POINT('Ctrl Pts',(8.2425464019257,-22.919371742163,85.3244857773327));
#60112=CARTESIAN_POINT('Ctrl Pts',(8.02456538963924,-23.1188689058929,85.2892109470019));
#60113=CARTESIAN_POINT('Ctrl Pts',(7.7276651131159,-23.3228372306943,85.2316907696594));
#60114=CARTESIAN_POINT('Ctrl Pts',(7.44619474014025,-23.4466175363318,85.1636679188582));
#60115=CARTESIAN_POINT('Ctrl Pts',(7.15762451622567,-23.5256490350712,85.081335317297));
#60116=CARTESIAN_POINT('Ctrl Pts',(6.91639948221045,-23.5617965035794,85.0042527237517));
#60117=CARTESIAN_POINT('Ctrl Pts',(6.61837867804194,-23.5621887278972,84.8958843854678));
#60118=CARTESIAN_POINT('Ctrl Pts',(6.33662733848544,-23.5123015142792,84.7785867703679));
#60119=CARTESIAN_POINT('Ctrl Pts',(5.97802318334561,-23.3851325798281,84.6119026529143));
#60120=CARTESIAN_POINT('Ctrl Pts',(5.63239849713251,-23.1599265610404,84.4265068018377));
#60121=CARTESIAN_POINT('Ctrl Pts',(5.39788990165802,-22.8921472712913,84.2833710814976));
#60122=CARTESIAN_POINT('Ctrl Pts',(5.23605135058215,-22.6488229062908,84.1801614493946));
#60123=CARTESIAN_POINT('Ctrl Pts',(5.0969095344909,-22.3790333101484,84.0874053636477));
#60124=CARTESIAN_POINT('Ctrl Pts',(4.9720724733076,-21.9635103030653,83.999566075602));
#60125=CARTESIAN_POINT('Ctrl Pts',(4.94371468395894,-21.6507340663161,83.9789798777728));
#60126=CARTESIAN_POINT('Ctrl Pts',(4.94371468395894,-21.5,83.9789798777728));
#60127=CARTESIAN_POINT('Ctrl Pts',(5.00120579598144,-21.5,83.9614679362901));
#60128=CARTESIAN_POINT('Ctrl Pts',(5.00120579598144,-21.3520059990089,83.9614679362901));
#60129=CARTESIAN_POINT('Ctrl Pts',(5.02938710354273,-21.0449379529334,83.9815481249973));
#60130=CARTESIAN_POINT('Ctrl Pts',(5.14210001521926,-20.6745440882475,84.0595031650574));
#60131=CARTESIAN_POINT('Ctrl Pts',(5.27274890176333,-20.4064934480325,84.1457116731447));
#60132=CARTESIAN_POINT('Ctrl Pts',(5.42805833516398,-20.1613379356766,84.2445019203697));
#60133=CARTESIAN_POINT('Ctrl Pts',(5.5842076611768,-19.9865699045241,84.3383374923964));
#60134=CARTESIAN_POINT('Ctrl Pts',(5.79518871998536,-19.8086662168602,84.4566186593402));
#60135=CARTESIAN_POINT('Ctrl Pts',(5.97008028592641,-19.6944825986058,84.5492829143672));
#60136=CARTESIAN_POINT('Ctrl Pts',(6.16024874649474,-19.6088242840925,84.6416704339889));
#60137=CARTESIAN_POINT('Ctrl Pts',(6.26265561097925,-19.5738308190456,84.6886756114093));
#60138=CARTESIAN_POINT('Ctrl Pts',(6.31228285326648,-19.5587773020503,84.7109583986528));
#60139=CARTESIAN_POINT('Ctrl Pts',(6.33718439395397,-19.5516405475664,84.7220307194513));
#60140=CARTESIAN_POINT('Ctrl Pts',(6.36638310919858,-19.5438854025941,84.7348502432122));
#60141=CARTESIAN_POINT('Ctrl Pts',(6.46664380786896,-19.5188490700099,84.7784451622438));
#60142=CARTESIAN_POINT('Ctrl Pts',(6.61214355835411,-19.4956974788605,84.8381010128625));
#60143=CARTESIAN_POINT('Ctrl Pts',(6.87934184713117,-19.4843021730789,84.9386886521805));
#60144=CARTESIAN_POINT('Ctrl Pts',(7.08098376058415,-19.5065990278365,85.0055173198125));
#60145=CARTESIAN_POINT('Ctrl Pts',(7.23572536065315,-19.5438603297829,85.0512669854069));
#60146=CARTESIAN_POINT('Ctrl Pts',(7.25902594561429,-19.5497685575946,85.0580779380141));
#60147=CARTESIAN_POINT('Ctrl Pts',(7.29398062082609,-19.5589776728157,85.068202640782));
#60148=CARTESIAN_POINT('Ctrl Pts',(7.37249143930395,-19.5818620333112,85.0903671757502));
#60149=CARTESIAN_POINT('Ctrl Pts',(7.47629543310783,-19.6184900161799,85.1180421488052));
#60150=CARTESIAN_POINT('Ctrl Pts',(7.61240028365782,-19.6768804536723,85.1519024555482));
#60151=CARTESIAN_POINT('Ctrl Pts',(7.7884588882969,-19.7679209606644,85.1922855511176));
#60152=CARTESIAN_POINT('Ctrl Pts',(8.00571902094384,-19.9161198082099,85.2354092037281));
#60153=CARTESIAN_POINT('Ctrl Pts',(8.20165416446568,-20.0945202553182,85.2681402867983));
#60154=CARTESIAN_POINT('Ctrl Pts',(8.33072651652134,-20.2441651242008,85.2867918154456));
#60155=CARTESIAN_POINT('Ctrl Pts',(8.45148795656648,-20.4072154069382,85.3028209480783));
#60156=CARTESIAN_POINT('Ctrl Pts',(8.57200758743931,-20.6057239697199,85.3169691524854));
#60157=CARTESIAN_POINT('Ctrl Pts',(8.69159825227611,-20.8958285905613,85.3288534467772));
#60158=CARTESIAN_POINT('Ctrl Pts',(8.75757356805284,-21.1735479434414,85.3346262878536));
#60159=CARTESIAN_POINT('Ctrl Pts',(8.77688460061852,-21.3763469753939,85.336233820364));
#60160=CARTESIAN_POINT('Ctrl Pts',(8.78059087654672,-21.5738186910076,85.3365468413902));
#60161=CARTESIAN_POINT('Ctrl Pts',(8.75630061671194,-21.9017339681359,85.334517176155));
#60162=CARTESIAN_POINT('Ctrl Pts',(8.65051985500575,-22.2305671395078,85.3253318026369));
#60163=CARTESIAN_POINT('Ctrl Pts',(8.50506066967912,-22.5045527127309,85.3091069381655));
#60164=CARTESIAN_POINT('Ctrl Pts',(8.39473328732379,-22.6791889660986,85.2957679284494));
#60165=CARTESIAN_POINT('Ctrl Pts',(8.21907518119456,-22.8898206522999,85.2710792257392));
#60166=CARTESIAN_POINT('Ctrl Pts',(8.00586508617554,-23.0837282560587,85.2354108414265));
#60167=CARTESIAN_POINT('Ctrl Pts',(7.71630377271468,-23.2813748438679,85.1780083266107));
#60168=CARTESIAN_POINT('Ctrl Pts',(7.44278857103648,-23.4008177940264,85.1110366251592));
#60169=CARTESIAN_POINT('Ctrl Pts',(7.16292149566871,-23.476956232333,85.0306247350017));
#60170=CARTESIAN_POINT('Ctrl Pts',(6.92920042935146,-23.5117274127833,84.9556727639564));
#60171=CARTESIAN_POINT('Ctrl Pts',(6.64052521451068,-23.5121075528597,84.8507009698725));
#60172=CARTESIAN_POINT('Ctrl Pts',(6.36728513118301,-23.4641122791779,84.7373259615023));
#60173=CARTESIAN_POINT('Ctrl Pts',(6.01870899323939,-23.3415395005,84.5762647242888));
#60174=CARTESIAN_POINT('Ctrl Pts',(5.68113207878283,-23.1237730049189,84.396893955329));
#60175=CARTESIAN_POINT('Ctrl Pts',(5.45052492150888,-22.8633215721594,84.2579345062791));
#60176=CARTESIAN_POINT('Ctrl Pts',(5.29094963212753,-22.6259977123551,84.1575892563859));
#60177=CARTESIAN_POINT('Ctrl Pts',(5.15335516091919,-22.362344512459,84.0672755210376));
#60178=CARTESIAN_POINT('Ctrl Pts',(5.02942559621785,-21.9550903286244,83.9815767221747));
#60179=CARTESIAN_POINT('Ctrl Pts',(5.00120579598144,-21.6479940009911,83.9614679362901));
#60180=CARTESIAN_POINT('Ctrl Pts',(5.00120579598144,-21.5,83.9614679362901));
#60181=CARTESIAN_POINT('',(4.82873245991394,-21.5,84.014003760738));
#60182=CARTESIAN_POINT('Origin',(9.31,-25.425,78.));
#60183=CARTESIAN_POINT('',(8.155,-25.5,78.));
#60184=CARTESIAN_POINT('Origin',(9.31,-25.5,78.));
#60185=CARTESIAN_POINT('',(8.305,-25.35,78.));
#60186=CARTESIAN_POINT('',(8.23,-25.425,78.));
#60187=CARTESIAN_POINT('Origin',(9.31,-25.35,78.));
#60188=CARTESIAN_POINT('Origin',(9.31,-24.485,78.));
#60189=CARTESIAN_POINT('',(10.0375846303818,-23.44,78.6932860921958));
#60190=CARTESIAN_POINT('',(8.30700212696576,-23.44,78.0634055730105));
#60191=CARTESIAN_POINT('Ctrl Pts',(10.0375846303818,-23.44,78.6932860921958));
#60192=CARTESIAN_POINT('Ctrl Pts',(9.96378821732871,-23.4632503226554,78.7707333921188));
#60193=CARTESIAN_POINT('Ctrl Pts',(9.78849047425474,-23.5225924173496,78.9050100514895));
#60194=CARTESIAN_POINT('Ctrl Pts',(9.51299812381197,-23.5976720228355,78.9966426113753));
#60195=CARTESIAN_POINT('Ctrl Pts',(9.27165366179481,-23.6401744298665,79.0099541241551));
#60196=CARTESIAN_POINT('Ctrl Pts',(9.08912965205693,-23.6586188959259,78.9859235830548));
#60197=CARTESIAN_POINT('Ctrl Pts',(8.92062369891718,-23.6619658680752,78.93222291379));
#60198=CARTESIAN_POINT('Ctrl Pts',(8.75994339020282,-23.6505635245521,78.8477059319911));
#60199=CARTESIAN_POINT('Ctrl Pts',(8.61580639791841,-23.6244291357707,78.7342228481503));
#60200=CARTESIAN_POINT('Ctrl Pts',(8.53710751827929,-23.5995950380918,78.6449366444775));
#60201=CARTESIAN_POINT('Ctrl Pts',(8.4893081082794,-23.5810512812345,78.5804189420813));
#60202=CARTESIAN_POINT('Ctrl Pts',(8.47679119967003,-23.5757772780198,78.5622829233047));
#60203=CARTESIAN_POINT('Ctrl Pts',(8.36906164076755,-23.5268334295508,78.3949081991338));
#60204=CARTESIAN_POINT('Ctrl Pts',(8.31739801874628,-23.4758129863659,78.2278557443297));
#60205=CARTESIAN_POINT('Ctrl Pts',(8.30700212696576,-23.44,78.0634055730105));
#60206=CARTESIAN_POINT('',(10.3129978730329,-23.4400000000023,77.9365944269688));
#60207=CARTESIAN_POINT('Origin',(9.31,-23.44,78.));
#60208=CARTESIAN_POINT('',(8.58241536963251,-23.4400000000023,77.3067139077891));
#60209=CARTESIAN_POINT('Ctrl Pts',(8.58241536961817,-23.44,77.3067139078042));
#60210=CARTESIAN_POINT('Ctrl Pts',(8.65618600625714,-23.4632422015298,77.2292936595168));
#60211=CARTESIAN_POINT('Ctrl Pts',(8.83158910154321,-23.522637422146,77.0950063597563));
#60212=CARTESIAN_POINT('Ctrl Pts',(9.10686435836405,-23.5977025591498,77.003294081653));
#60213=CARTESIAN_POINT('Ctrl Pts',(9.34839642462173,-23.6401800947028,76.9900977598095));
#60214=CARTESIAN_POINT('Ctrl Pts',(9.54592789251119,-23.6601491700001,77.0161150091369));
#60215=CARTESIAN_POINT('Ctrl Pts',(9.71319142839158,-23.6616254923616,77.0735905656994));
#60216=CARTESIAN_POINT('Ctrl Pts',(9.92566013575099,-23.644055915951,77.1912681046098));
#60217=CARTESIAN_POINT('Ctrl Pts',(10.0483680006109,-23.6129990647924,77.3084577996669));
#60218=CARTESIAN_POINT('Ctrl Pts',(10.1306989862535,-23.5810249250644,77.4196554703819));
#60219=CARTESIAN_POINT('Ctrl Pts',(10.1432239502022,-23.5757515322204,77.4377948245863));
#60220=CARTESIAN_POINT('Ctrl Pts',(10.2509072559687,-23.5268295608697,77.6050981709781));
#60221=CARTESIAN_POINT('Ctrl Pts',(10.3026077290777,-23.4757931855883,77.7722351791483));
#60222=CARTESIAN_POINT('Ctrl Pts',(10.3129978730342,-23.44,77.9365944269895));
#60223=CARTESIAN_POINT('',(8.305,-23.44,78.));
#60224=CARTESIAN_POINT('Origin',(9.31,-23.44,78.));
#60225=CARTESIAN_POINT('',(8.305,-24.485,78.));
#60226=CARTESIAN_POINT('Origin',(9.31,-23.44,78.));
#60227=CARTESIAN_POINT('Origin',(9.31,-25.5,78.));
#60228=CARTESIAN_POINT('',(2.01,-25.5,78.));
#60229=CARTESIAN_POINT('Origin',(9.31,-25.5,78.));
#60230=CARTESIAN_POINT('Ctrl Pts',(10.100212007486,-23.2297865267127,78.8219759032923));
#60231=CARTESIAN_POINT('Ctrl Pts',(10.0103245365164,-23.2613499461505,78.912999905046));
#60232=CARTESIAN_POINT('Ctrl Pts',(9.80443306533852,-23.339235126355,79.0610556336041));
#60233=CARTESIAN_POINT('Ctrl Pts',(9.50086601864425,-23.4330668442817,79.1505987981109));
#60234=CARTESIAN_POINT('Ctrl Pts',(9.24114419357868,-23.4856018928221,79.1585650126785));
#60235=CARTESIAN_POINT('Ctrl Pts',(9.04620851329942,-23.5082837204292,79.1299209668847));
#60236=CARTESIAN_POINT('Ctrl Pts',(8.86630044007771,-23.5123967187664,79.0720196330274));
#60237=CARTESIAN_POINT('Ctrl Pts',(8.69364486134355,-23.4983842652002,78.9832904164185));
#60238=CARTESIAN_POINT('Ctrl Pts',(8.53662363166247,-23.4661751204574,78.8648197598721));
#60239=CARTESIAN_POINT('Ctrl Pts',(8.4489747625146,-23.4353586041831,78.7708091230029));
#60240=CARTESIAN_POINT('Ctrl Pts',(8.39503262461223,-23.4122040782005,78.7021958553138));
#60241=CARTESIAN_POINT('Ctrl Pts',(8.38081350063257,-23.4055972563583,78.6828313686353));
#60242=CARTESIAN_POINT('Ctrl Pts',(8.2578365866536,-23.3442373462283,78.5034801846723));
#60243=CARTESIAN_POINT('Ctrl Pts',(8.19224688382286,-23.2784043599677,78.3181334130021));
#60244=CARTESIAN_POINT('Ctrl Pts',(8.17630655668227,-23.2297865267127,78.1217315856572));
#60245=CARTESIAN_POINT('Ctrl Pts',(10.0793362151179,-23.2998576844751,78.7790792995935));
#60246=CARTESIAN_POINT('Ctrl Pts',(9.99485230101193,-23.3286228262624,78.8655473612077));
#60247=CARTESIAN_POINT('Ctrl Pts',(9.79910201738819,-23.4003640892565,79.009055802932));
#60248=CARTESIAN_POINT('Ctrl Pts',(9.50491384035135,-23.4879249343831,79.0992633727804));
#60249=CARTESIAN_POINT('Ctrl Pts',(9.25130749167517,-23.5371227532837,79.1090171864575));
#60250=CARTESIAN_POINT('Ctrl Pts',(9.06051438646356,-23.5583916441821,79.0819108022503));
#60251=CARTESIAN_POINT('Ctrl Pts',(8.88441470298779,-23.5622512059598,79.0254124040774));
#60252=CARTESIAN_POINT('Ctrl Pts',(8.71574308357439,-23.5491044557046,78.938087008499));
#60253=CARTESIAN_POINT('Ctrl Pts',(8.56302183467341,-23.5189230023405,78.8212783528971));
#60254=CARTESIAN_POINT('Ctrl Pts',(8.47834776994348,-23.4900971027019,78.7288410132963));
#60255=CARTESIAN_POINT('Ctrl Pts',(8.42645705160579,-23.4684807083556,78.6615934910345));
#60256=CARTESIAN_POINT('Ctrl Pts',(8.41280930323009,-23.462321544408,78.6426422389549));
#60257=CARTESIAN_POINT('Ctrl Pts',(8.29488073666906,-23.4050771273758,78.4672608815071));
#60258=CARTESIAN_POINT('Ctrl Pts',(8.23391095961167,-23.3441519573982,78.2879642490827));
#60259=CARTESIAN_POINT('Ctrl Pts',(8.21987174677676,-23.2998576844751,78.1022895814417));
#60260=CARTESIAN_POINT('Ctrl Pts',(10.0584604227499,-23.3699288422376,78.7361826958946));
#60261=CARTESIAN_POINT('Ctrl Pts',(9.97926045283321,-23.3959774425435,78.8181859359572));
#60262=CARTESIAN_POINT('Ctrl Pts',(9.79382152220507,-23.4614634544481,78.9570098821616));
#60263=CARTESIAN_POINT('Ctrl Pts',(9.50895030210486,-23.5428139327341,79.0479780367058));
#60264=CARTESIAN_POINT('Ctrl Pts',(9.26149036369832,-23.5886535694049,79.0595019503761));
#60265=CARTESIAN_POINT('Ctrl Pts',(9.07482377889279,-23.608510972173,79.0339337476891));
#60266=CARTESIAN_POINT('Ctrl Pts',(8.9025094360071,-23.6121113808818,78.97883014274));
#60267=CARTESIAN_POINT('Ctrl Pts',(8.73784516797198,-23.5998433340478,78.8929093399106));
#60268=CARTESIAN_POINT('Ctrl Pts',(8.58940819490746,-23.5716812538877,78.7777642551252));
#60269=CARTESIAN_POINT('Ctrl Pts',(8.50773451085042,-23.5448565395729,78.6869047541841));
#60270=CARTESIAN_POINT('Ctrl Pts',(8.45788368128585,-23.5247746510794,78.6210213063607));
#60271=CARTESIAN_POINT('Ctrl Pts',(8.44479539707251,-23.5190529899701,78.602472052985));
#60272=CARTESIAN_POINT('Ctrl Pts',(8.3320174907521,-23.4659936484033,78.431127502299));
#60273=CARTESIAN_POINT('Ctrl Pts',(8.27573394295747,-23.4100653889354,78.2580249082491));
#60274=CARTESIAN_POINT('Ctrl Pts',(8.26343693687126,-23.3699288422376,78.0828475772261));
#60275=CARTESIAN_POINT('Ctrl Pts',(10.0375846303818,-23.44,78.6932860921958));
#60276=CARTESIAN_POINT('Ctrl Pts',(9.96378821732871,-23.4632503226554,78.7707333921188));
#60277=CARTESIAN_POINT('Ctrl Pts',(9.78849047425474,-23.5225924173496,78.9050100514895));
#60278=CARTESIAN_POINT('Ctrl Pts',(9.51299812381197,-23.5976720228355,78.9966426113753));
#60279=CARTESIAN_POINT('Ctrl Pts',(9.27165366179481,-23.6401744298665,79.0099541241551));
#60280=CARTESIAN_POINT('Ctrl Pts',(9.08912965205693,-23.6586188959259,78.9859235830548));
#60281=CARTESIAN_POINT('Ctrl Pts',(8.92062369891718,-23.6619658680752,78.93222291379));
#60282=CARTESIAN_POINT('Ctrl Pts',(8.75994339020282,-23.6505635245521,78.8477059319911));
#60283=CARTESIAN_POINT('Ctrl Pts',(8.61580639791841,-23.6244291357707,78.7342228481503));
#60284=CARTESIAN_POINT('Ctrl Pts',(8.53710751827929,-23.5995950380918,78.6449366444775));
#60285=CARTESIAN_POINT('Ctrl Pts',(8.4893081082794,-23.5810512812345,78.5804189420813));
#60286=CARTESIAN_POINT('Ctrl Pts',(8.47679119967003,-23.5757772780198,78.5622829233047));
#60287=CARTESIAN_POINT('Ctrl Pts',(8.36906164076755,-23.5268334295508,78.3949081991338));
#60288=CARTESIAN_POINT('Ctrl Pts',(8.31739801874628,-23.4758129863659,78.2278557443297));
#60289=CARTESIAN_POINT('Ctrl Pts',(8.30700212696576,-23.44,78.0634055730105));
#60290=CARTESIAN_POINT('Ctrl Pts',(10.0375846303818,-23.44,78.6932860921958));
#60291=CARTESIAN_POINT('Ctrl Pts',(9.9599378066044,-23.44,78.7997428949848));
#60292=CARTESIAN_POINT('Ctrl Pts',(9.86722691076642,-23.44,78.8961653627146));
#60293=CARTESIAN_POINT('Ctrl Pts',(9.66852004688849,-23.44,79.0475540438521));
#60294=CARTESIAN_POINT('Ctrl Pts',(9.56417005974731,-23.44,79.106184738785));
#60295=CARTESIAN_POINT('Ctrl Pts',(9.45276488839657,-23.44,79.1451885759221));
#60296=CARTESIAN_POINT('Ctrl Pts',(8.46452272321397,-23.44,78.7854978435489));
#60297=CARTESIAN_POINT('Ctrl Pts',(8.42330536322784,-23.44,78.716092159532));
#60298=CARTESIAN_POINT('Ctrl Pts',(8.39052202042233,-23.44,78.6417586933716));
#60299=CARTESIAN_POINT('Ctrl Pts',(8.31364989985943,-23.44,78.4045407779282));
#60300=CARTESIAN_POINT('Ctrl Pts',(8.29551551211911,-23.44,78.2321594268118));
#60301=CARTESIAN_POINT('Ctrl Pts',(8.30700212696576,-23.44,78.0634055730105));
#60302=CARTESIAN_POINT('Ctrl Pts',(8.519787992514,-23.2297865267127,77.1780240967077));
#60303=CARTESIAN_POINT('Ctrl Pts',(8.60964406660961,-23.2613389213359,77.0870318888077));
#60304=CARTESIAN_POINT('Ctrl Pts',(8.81560969574407,-23.339249297738,76.9390093127447));
#60305=CARTESIAN_POINT('Ctrl Pts',(9.11896640120719,-23.4330872349703,76.8493596419297));
#60306=CARTESIAN_POINT('Ctrl Pts',(9.3788902833647,-23.4855876966743,76.8415124408269));
#60307=CARTESIAN_POINT('Ctrl Pts',(9.58984999260555,-23.5101434522743,76.872532168987));
#60308=CARTESIAN_POINT('Ctrl Pts',(9.76844966013923,-23.5119591404095,76.9341462709327));
#60309=CARTESIAN_POINT('Ctrl Pts',(9.99707390435989,-23.4903522775185,77.0575739991169));
#60310=CARTESIAN_POINT('Ctrl Pts',(10.1320938555494,-23.4520581358879,77.1796744771316));
#60311=CARTESIAN_POINT('Ctrl Pts',(10.2250132495704,-23.412138947756,77.2979250401662));
#60312=CARTESIAN_POINT('Ctrl Pts',(10.2392416738491,-23.4055315301041,77.3172947002189));
#60313=CARTESIAN_POINT('Ctrl Pts',(10.3621589089987,-23.3442025877036,77.496565902309));
#60314=CARTESIAN_POINT('Ctrl Pts',(10.427761929485,-23.2783774794697,77.681975176348));
#60315=CARTESIAN_POINT('Ctrl Pts',(10.4436934433177,-23.2297865267127,77.8782684143427));
#60316=CARTESIAN_POINT('Ctrl Pts',(8.54066378488206,-23.2998576844752,77.2209207004065));
#60317=CARTESIAN_POINT('Ctrl Pts',(8.62510929439727,-23.3286069304059,77.1344916746785));
#60318=CARTESIAN_POINT('Ctrl Pts',(8.8209342962108,-23.4003746742759,76.9910095890714));
#60319=CARTESIAN_POINT('Ctrl Pts',(9.11491770383446,-23.4879441141189,76.9006932924059));
#60320=CARTESIAN_POINT('Ctrl Pts',(9.36872278502232,-23.5371069494853,76.8910608603316));
#60321=CARTESIAN_POINT('Ctrl Pts',(9.57520010070161,-23.5601348424691,76.9204112874013));
#60322=CARTESIAN_POINT('Ctrl Pts',(9.75002742645247,-23.56183762232,76.9806466551884));
#60323=CARTESIAN_POINT('Ctrl Pts',(9.97326596229238,-23.5415767678213,77.1021600329057));
#60324=CARTESIAN_POINT('Ctrl Pts',(10.1042121603643,-23.5056801367365,77.222624707157));
#60325=CARTESIAN_POINT('Ctrl Pts',(10.1935880244434,-23.4684159698535,77.3385282257988));
#60326=CARTESIAN_POINT('Ctrl Pts',(10.2072463553255,-23.462255399493,77.3574841605641));
#60327=CARTESIAN_POINT('Ctrl Pts',(10.3251091704039,-23.4050474225909,77.5327786005297));
#60328=CARTESIAN_POINT('Ctrl Pts',(10.3861102406279,-23.3441130561887,77.7121608586934));
#60329=CARTESIAN_POINT('Ctrl Pts',(10.4001282532232,-23.2998576844752,77.8977104185583));
#60330=CARTESIAN_POINT('Ctrl Pts',(8.56153957725011,-23.3699288422376,77.2638173041054));
#60331=CARTESIAN_POINT('Ctrl Pts',(8.64072077846948,-23.3959741924597,77.1818338736461));
#60332=CARTESIAN_POINT('Ctrl Pts',(8.82626450107649,-23.4615120456081,77.0430060834296));
#60333=CARTESIAN_POINT('Ctrl Pts',(9.11091305573679,-23.5428456800012,76.9519604311767));
#60334=CARTESIAN_POINT('Ctrl Pts',(9.35856392296411,-23.5886608418917,76.9405493403047));
#60335=CARTESIAN_POINT('Ctrl Pts',(9.56057778441512,-23.6101577798053,76.9682358907225));
#60336=CARTESIAN_POINT('Ctrl Pts',(9.73161366207835,-23.611747010451,77.0270901814438));
#60337=CARTESIAN_POINT('Ctrl Pts',(9.9494680778185,-23.5928314256482,77.146682070821));
#60338=CARTESIAN_POINT('Ctrl Pts',(10.0762496957961,-23.5593770639438,77.2655075696414));
#60339=CARTESIAN_POINT('Ctrl Pts',(10.1621242113804,-23.5247479029669,77.3790522847493));
#60340=CARTESIAN_POINT('Ctrl Pts',(10.1752192687258,-23.5190276628316,77.3976053642411));
#60341=CARTESIAN_POINT('Ctrl Pts',(10.2879569945636,-23.4659847259824,77.5688854727573));
#60342=CARTESIAN_POINT('Ctrl Pts',(10.3442594179347,-23.4100576088693,77.742049496803));
#60343=CARTESIAN_POINT('Ctrl Pts',(10.3565630631287,-23.3699288422376,77.9171524227739));
#60344=CARTESIAN_POINT('Ctrl Pts',(8.58241536961817,-23.44,77.3067139078042));
#60345=CARTESIAN_POINT('Ctrl Pts',(8.65618600625714,-23.4632422015298,77.2292936595168));
#60346=CARTESIAN_POINT('Ctrl Pts',(8.83158910154321,-23.522637422146,77.0950063597563));
#60347=CARTESIAN_POINT('Ctrl Pts',(9.10686435836405,-23.5977025591498,77.003294081653));
#60348=CARTESIAN_POINT('Ctrl Pts',(9.34839642462173,-23.6401800947028,76.9900977598095));
#60349=CARTESIAN_POINT('Ctrl Pts',(9.54592789251119,-23.6601491700001,77.0161150091369));
#60350=CARTESIAN_POINT('Ctrl Pts',(9.71319142839158,-23.6616254923616,77.0735905656994));
#60351=CARTESIAN_POINT('Ctrl Pts',(9.92566013575099,-23.644055915951,77.1912681046098));
#60352=CARTESIAN_POINT('Ctrl Pts',(10.0483680006109,-23.6129990647924,77.3084577996669));
#60353=CARTESIAN_POINT('Ctrl Pts',(10.1306989862535,-23.5810249250644,77.4196554703819));
#60354=CARTESIAN_POINT('Ctrl Pts',(10.1432239502022,-23.5757515322204,77.4377948245863));
#60355=CARTESIAN_POINT('Ctrl Pts',(10.2509072559687,-23.5268295608697,77.6050981709781));
#60356=CARTESIAN_POINT('Ctrl Pts',(10.3026077290777,-23.4757931855883,77.7722351791483));
#60357=CARTESIAN_POINT('Ctrl Pts',(10.3129978730342,-23.44,77.9365944269895));
#60358=CARTESIAN_POINT('Ctrl Pts',(8.58241536961817,-23.44,77.3067139078042));
#60359=CARTESIAN_POINT('Ctrl Pts',(8.66006016612818,-23.44,77.2002598844773));
#60360=CARTESIAN_POINT('Ctrl Pts',(8.75276823603309,-23.44,77.1038396887893));
#60361=CARTESIAN_POINT('Ctrl Pts',(8.95147388732374,-23.44,76.9524493606504));
#60362=CARTESIAN_POINT('Ctrl Pts',(9.05582670211928,-23.44,76.8938163949113));
#60363=CARTESIAN_POINT('Ctrl Pts',(9.16723511160343,-23.44,76.8548114240778));
#60364=CARTESIAN_POINT('Ctrl Pts',(10.155477276786,-23.44,77.2145021564511));
#60365=CARTESIAN_POINT('Ctrl Pts',(10.1966868174929,-23.44,77.283894673627));
#60366=CARTESIAN_POINT('Ctrl Pts',(10.229465540476,-23.44,77.3582131109841));
#60367=CARTESIAN_POINT('Ctrl Pts',(10.3063468190756,-23.44,77.5954278309571));
#60368=CARTESIAN_POINT('Ctrl Pts',(10.3244855296182,-23.44,77.7678252686633));
#60369=CARTESIAN_POINT('Ctrl Pts',(10.3129978730342,-23.44,77.9365944269895));
#60370=CARTESIAN_POINT('Ctrl Pts',(12.1440294707702,-15.3457361617732,78.9916063779574));
#60371=CARTESIAN_POINT('Ctrl Pts',(12.0821287866527,-15.3383729044183,79.1685196844361));
#60372=CARTESIAN_POINT('Ctrl Pts',(11.9811196883727,-15.4003238547929,79.3825863055803));
#60373=CARTESIAN_POINT('Ctrl Pts',(11.8251071448527,-15.616984349081,79.6451820555524));
#60374=CARTESIAN_POINT('Ctrl Pts',(11.6852150750259,-15.9157775367878,79.8401596355449));
#60375=CARTESIAN_POINT('Ctrl Pts',(11.6322385355776,-16.4531466810754,79.9023659741719));
#60376=CARTESIAN_POINT('Ctrl Pts',(11.7419583042977,-16.8055520460372,79.7657541392426));
#60377=CARTESIAN_POINT('Ctrl Pts',(11.822863335852,-16.9636835154004,79.6436043679924));
#60378=CARTESIAN_POINT('Ctrl Pts',(11.8340060584782,-16.9839356481672,79.626485701499));
#60379=CARTESIAN_POINT('Ctrl Pts',(11.8910343120941,-17.0804741647385,79.5365456795022));
#60380=CARTESIAN_POINT('Ctrl Pts',(11.9963709991369,-17.2117774433501,79.3562680459212));
#60381=CARTESIAN_POINT('Ctrl Pts',(12.0925286612292,-17.2551291983681,79.1341301729733));
#60382=CARTESIAN_POINT('Ctrl Pts',(12.1731938226851,-17.2549658653676,78.9122669584772));
#60383=CARTESIAN_POINT('Ctrl Pts',(12.228036692318,-17.218306148821,78.7260201971924));
#60384=CARTESIAN_POINT('Ctrl Pts',(12.2717094191553,-17.0934753320961,78.5017481928062));
#60385=CARTESIAN_POINT('Ctrl Pts',(12.2987015121157,-16.9349741098207,78.3119581382534));
#60386=CARTESIAN_POINT('Ctrl Pts',(12.3081423262004,-16.7295975635937,78.172212569198));
#60387=CARTESIAN_POINT('Ctrl Pts',(12.3111010412262,-16.492435283584,78.0968890708661));
#60388=CARTESIAN_POINT('Ctrl Pts',(12.3115831055068,-16.2454177966105,78.0700185886829));
#60389=CARTESIAN_POINT('Ctrl Pts',(12.3106379014819,-15.9361493339683,78.1306696064297));
#60390=CARTESIAN_POINT('Ctrl Pts',(12.2972420283652,-15.6231316758572,78.3377707078825));
#60391=CARTESIAN_POINT('Ctrl Pts',(12.2499737983051,-15.4084011027765,78.6408069135594));
#60392=CARTESIAN_POINT('Ctrl Pts',(12.1846480803193,-15.3505678575739,78.8755176364136));
#60393=CARTESIAN_POINT('Ctrl Pts',(12.1440294707702,-15.3457361617732,78.9916063779574));
#60394=CARTESIAN_POINT('Ctrl Pts',(12.1905411751434,-15.395718781424,79.0100646834078));
#60395=CARTESIAN_POINT('Ctrl Pts',(12.1307865477481,-15.3884188195122,79.1802503183488));
#60396=CARTESIAN_POINT('Ctrl Pts',(12.0347735529135,-15.4494252933908,79.3861988883646));
#60397=CARTESIAN_POINT('Ctrl Pts',(11.8885687474473,-15.6581438008607,79.636587449847));
#60398=CARTESIAN_POINT('Ctrl Pts',(11.7598527815262,-15.9428103951435,79.8196635436855));
#60399=CARTESIAN_POINT('Ctrl Pts',(11.7123017216896,-16.4419422338359,79.8765562283324));
#60400=CARTESIAN_POINT('Ctrl Pts',(11.8116717647762,-16.7724433312399,79.7503244727558));
#60401=CARTESIAN_POINT('Ctrl Pts',(11.8868691413704,-16.9237865974938,79.6346407897848));
#60402=CARTESIAN_POINT('Ctrl Pts',(11.8971829796672,-16.9430695195421,79.618457434879));
#60403=CARTESIAN_POINT('Ctrl Pts',(11.9502752858818,-17.0355212070356,79.5331286750323));
#60404=CARTESIAN_POINT('Ctrl Pts',(12.0491364656578,-17.1626660611137,79.3609572273587));
#60405=CARTESIAN_POINT('Ctrl Pts',(12.1410059087477,-17.2051327276356,79.1471173412086));
#60406=CARTESIAN_POINT('Ctrl Pts',(12.2185735988939,-17.2049790741984,78.9337592374503));
#60407=CARTESIAN_POINT('Ctrl Pts',(12.2718391220554,-17.1690378747736,78.7548462589905));
#60408=CARTESIAN_POINT('Ctrl Pts',(12.3149022681015,-17.0481569211274,78.5414316970799));
#60409=CARTESIAN_POINT('Ctrl Pts',(12.3419162375973,-16.89588396213,78.3621822312909));
#60410=CARTESIAN_POINT('Ctrl Pts',(12.3519442672886,-16.7012080271386,78.2321915109205));
#60411=CARTESIAN_POINT('Ctrl Pts',(12.3553529574687,-16.4792730984203,78.1627644017751));
#60412=CARTESIAN_POINT('Ctrl Pts',(12.3560377852108,-16.2491700223592,78.1381695110903));
#60413=CARTESIAN_POINT('Ctrl Pts',(12.3546266916132,-15.9610344808616,78.1936295942804));
#60414=CARTESIAN_POINT('Ctrl Pts',(12.3403320117296,-15.6644959222293,78.3860774975201));
#60415=CARTESIAN_POINT('Ctrl Pts',(12.2932391850083,-15.4570233754469,78.673215845813));
#60416=CARTESIAN_POINT('Ctrl Pts',(12.2296649765981,-15.4004233493121,78.8984274812488));
#60417=CARTESIAN_POINT('Ctrl Pts',(12.1905411751434,-15.395718781424,79.0100646834078));
#60418=CARTESIAN_POINT('Ctrl Pts',(12.2370528795166,-15.4457014010748,79.0285229888583));
#60419=CARTESIAN_POINT('Ctrl Pts',(12.1798257226226,-15.4387970155116,79.1916890394376));
#60420=CARTESIAN_POINT('Ctrl Pts',(12.0884081621552,-15.4985468621786,79.3898292947456));
#60421=CARTESIAN_POINT('Ctrl Pts',(11.9522340660948,-15.6994288658102,79.6278251275205));
#60422=CARTESIAN_POINT('Ctrl Pts',(11.834568849452,-15.9701317113529,79.7991100429138));
#60423=CARTESIAN_POINT('Ctrl Pts',(11.7920587468212,-16.4301848099057,79.8510263063962));
#60424=CARTESIAN_POINT('Ctrl Pts',(11.8815772239625,-16.7400260169906,79.7347243019166));
#60425=CARTESIAN_POINT('Ctrl Pts',(11.9506563012613,-16.883501785339,79.6258869212831));
#60426=CARTESIAN_POINT('Ctrl Pts',(11.9602409595347,-16.9020175268376,79.6105578504383));
#60427=CARTESIAN_POINT('Ctrl Pts',(12.0094076680351,-16.9904823469893,79.5297823783282));
#60428=CARTESIAN_POINT('Ctrl Pts',(12.1018520459692,-17.1134311038727,79.3657191698453));
#60429=CARTESIAN_POINT('Ctrl Pts',(12.1894185541784,-17.1550573199279,79.1601685949679));
#60430=CARTESIAN_POINT('Ctrl Pts',(12.2639231573512,-17.1548908469061,78.9552998254218));
#60431=CARTESIAN_POINT('Ctrl Pts',(12.3155809210026,-17.1197507947583,78.783714952818));
#60432=CARTESIAN_POINT('Ctrl Pts',(12.3580545728541,-17.0027799265832,78.5811277203043));
#60433=CARTESIAN_POINT('Ctrl Pts',(12.3850999349634,-16.8567601611705,78.412439808554));
#60434=CARTESIAN_POINT('Ctrl Pts',(12.395719201828,-16.6728435871762,78.2921907493411));
#60435=CARTESIAN_POINT('Ctrl Pts',(12.3995908338668,-16.4661177374306,78.2286929082959));
#60436=CARTESIAN_POINT('Ctrl Pts',(12.4004721034329,-16.2529370512118,78.2063226605274));
#60437=CARTESIAN_POINT('Ctrl Pts',(12.3986099640282,-15.9858739114076,78.2566551537243));
#60438=CARTESIAN_POINT('Ctrl Pts',(12.3834130133868,-15.7059406852543,78.4344048281252));
#60439=CARTESIAN_POINT('Ctrl Pts',(12.3364987711348,-15.5056308812999,78.7056068063562));
#60440=CARTESIAN_POINT('Ctrl Pts',(12.2746913544106,-15.4503175838733,78.921418150445));
#60441=CARTESIAN_POINT('Ctrl Pts',(12.2370528795166,-15.4457014010748,79.0285229888583));
#60442=CARTESIAN_POINT('Ctrl Pts',(12.2835645838897,-15.4956840207256,79.0469812943087));
#60443=CARTESIAN_POINT('Ctrl Pts',(12.228483483718,-15.4888429306054,79.2034196733504));
#60444=CARTESIAN_POINT('Ctrl Pts',(12.1420620266961,-15.5476483007766,79.3934418775299));
#60445=CARTESIAN_POINT('Ctrl Pts',(12.0156956686893,-15.7405883175899,79.6192305218151));
#60446=CARTESIAN_POINT('Ctrl Pts',(11.9092065559523,-15.9971645697086,79.7786139510543));
#60447=CARTESIAN_POINT('Ctrl Pts',(11.8721219329333,-16.4189803626662,79.8252165605567));
#60448=CARTESIAN_POINT('Ctrl Pts',(11.951290684441,-16.7069173021933,79.7192946354299));
#60449=CARTESIAN_POINT('Ctrl Pts',(12.0146621067797,-16.8436048674325,79.6169233430755));
#60450=CARTESIAN_POINT('Ctrl Pts',(12.0234178807236,-16.8611513982124,79.6025295838183));
#60451=CARTESIAN_POINT('Ctrl Pts',(12.0686486418228,-16.9455293892864,79.5263653738583));
#60452=CARTESIAN_POINT('Ctrl Pts',(12.1546175124901,-17.0643197216363,79.3704083512828));
#60453=CARTESIAN_POINT('Ctrl Pts',(12.2378958016969,-17.1050608491954,79.1731557632031));
#60454=CARTESIAN_POINT('Ctrl Pts',(12.3093029335599,-17.1049040557369,78.9767921043949));
#60455=CARTESIAN_POINT('Ctrl Pts',(12.35938335074,-17.0704825207109,78.8125410146161));
#60456=CARTESIAN_POINT('Ctrl Pts',(12.4012474218003,-16.9574615156145,78.620811224578));
#60457=CARTESIAN_POINT('Ctrl Pts',(12.4283146604451,-16.8176700134799,78.4626639015916));
#60458=CARTESIAN_POINT('Ctrl Pts',(12.4395211429162,-16.6444540507211,78.3521696910637));
#60459=CARTESIAN_POINT('Ctrl Pts',(12.4438427501093,-16.4529555522669,78.2945682392049));
#60460=CARTESIAN_POINT('Ctrl Pts',(12.444926783137,-16.2566892769605,78.2744735829348));
#60461=CARTESIAN_POINT('Ctrl Pts',(12.4425987541595,-16.010759058301,78.319615141575));
#60462=CARTESIAN_POINT('Ctrl Pts',(12.4265029967512,-15.7473049316263,78.4827116177628));
#60463=CARTESIAN_POINT('Ctrl Pts',(12.379764157838,-15.5542531539703,78.7380157386097));
#60464=CARTESIAN_POINT('Ctrl Pts',(12.3197082506894,-15.5001730756115,78.9443279952801));
#60465=CARTESIAN_POINT('Ctrl Pts',(12.2835645838897,-15.4956840207256,79.0469812943087));
#60466=CARTESIAN_POINT('',(12.1440294707702,-15.3457361617732,78.9916063779574));
#60467=CARTESIAN_POINT('',(12.2835645838897,-15.4956840207256,79.0469812943087));
#60468=CARTESIAN_POINT('',(12.1440294707702,-15.3457361617732,78.9916063779574));
#60469=CARTESIAN_POINT('',(12.4444120815709,-16.3000163632569,78.2841628434877));
#60470=CARTESIAN_POINT('Ctrl Pts',(12.2835645838897,-15.4956840207256,79.0469812943087));
#60471=CARTESIAN_POINT('Ctrl Pts',(12.228483483718,-15.4888429306054,79.2034196733504));
#60472=CARTESIAN_POINT('Ctrl Pts',(12.1420620266961,-15.5476483007766,79.3934418775299));
#60473=CARTESIAN_POINT('Ctrl Pts',(12.0156956686893,-15.7405883175899,79.6192305218151));
#60474=CARTESIAN_POINT('Ctrl Pts',(11.9092065559523,-15.9971645697086,79.7786139510543));
#60475=CARTESIAN_POINT('Ctrl Pts',(11.8721219329333,-16.4189803626662,79.8252165605567));
#60476=CARTESIAN_POINT('Ctrl Pts',(11.951290684441,-16.7069173021933,79.7192946354299));
#60477=CARTESIAN_POINT('Ctrl Pts',(12.0146621067797,-16.8436048674325,79.6169233430755));
#60478=CARTESIAN_POINT('Ctrl Pts',(12.0234178807236,-16.8611513982124,79.6025295838183));
#60479=CARTESIAN_POINT('Ctrl Pts',(12.0686486418228,-16.9455293892864,79.5263653738583));
#60480=CARTESIAN_POINT('Ctrl Pts',(12.1546175124901,-17.0643197216363,79.3704083512828));
#60481=CARTESIAN_POINT('Ctrl Pts',(12.2378958016969,-17.1050608491954,79.1731557632031));
#60482=CARTESIAN_POINT('Ctrl Pts',(12.3093029335599,-17.1049040557369,78.9767921043949));
#60483=CARTESIAN_POINT('Ctrl Pts',(12.35938335074,-17.0704825207109,78.8125410146161));
#60484=CARTESIAN_POINT('Ctrl Pts',(12.4012474218003,-16.9574615156145,78.620811224578));
#60485=CARTESIAN_POINT('Ctrl Pts',(12.4283146604451,-16.8176700134799,78.4626639015916));
#60486=CARTESIAN_POINT('Ctrl Pts',(12.4395211429162,-16.6444540507211,78.3521696910637));
#60487=CARTESIAN_POINT('Ctrl Pts',(12.4438427501093,-16.4529555522669,78.2945682392049));
#60488=CARTESIAN_POINT('Ctrl Pts',(12.4443952514524,-16.3529241160095,78.2843265544088));
#60489=CARTESIAN_POINT('Ctrl Pts',(12.4444118401433,-16.3019162824862,78.2841619672088));
#60490=CARTESIAN_POINT('Ctrl Pts',(12.4444120815709,-16.3000163632569,78.2841628434877));
#60491=CARTESIAN_POINT('Ctrl Pts',(12.4444120815709,-16.3000163632569,78.2841628434877));
#60492=CARTESIAN_POINT('Ctrl Pts',(12.4444243208177,-16.2036993661096,78.2842072667228));
#60493=CARTESIAN_POINT('Ctrl Pts',(12.442494968104,-16.0090602960789,78.3206667938524));
#60494=CARTESIAN_POINT('Ctrl Pts',(12.4265029967512,-15.7473049316263,78.4827116177628));
#60495=CARTESIAN_POINT('Ctrl Pts',(12.379764157838,-15.5542531539703,78.7380157386097));
#60496=CARTESIAN_POINT('Ctrl Pts',(12.3197082506894,-15.5001730756115,78.9443279952801));
#60497=CARTESIAN_POINT('Ctrl Pts',(12.2835645838897,-15.4956840207256,79.0469812943087));
#60498=CARTESIAN_POINT('',(12.2711805139213,-17.0828938614663,78.4968565980093));
#60499=CARTESIAN_POINT('Ctrl Pts',(12.1440294707702,-15.3457361617732,78.9916063779574));
#60500=CARTESIAN_POINT('Ctrl Pts',(12.1846480803193,-15.3505678575739,78.8755176364136));
#60501=CARTESIAN_POINT('Ctrl Pts',(12.2499737983051,-15.4084011027765,78.6408069135594));
#60502=CARTESIAN_POINT('Ctrl Pts',(12.2972420283652,-15.6231316758572,78.3377707078825));
#60503=CARTESIAN_POINT('Ctrl Pts',(12.3106379014819,-15.9361493339683,78.1306696064297));
#60504=CARTESIAN_POINT('Ctrl Pts',(12.3115831055068,-16.2454177966105,78.0700185886829));
#60505=CARTESIAN_POINT('Ctrl Pts',(12.3111010412262,-16.492435283584,78.0968890708661));
#60506=CARTESIAN_POINT('Ctrl Pts',(12.3081423262004,-16.7295975635937,78.172212569198));
#60507=CARTESIAN_POINT('Ctrl Pts',(12.2988420797468,-16.9319161855434,78.3098774168852));
#60508=CARTESIAN_POINT('Ctrl Pts',(12.2792560441049,-17.0491162087367,78.4486637689));
#60509=CARTESIAN_POINT('Ctrl Pts',(12.2711805139213,-17.0828938614663,78.4968565980093));
#60510=CARTESIAN_POINT('',(11.8979359134617,-17.0829544530057,79.5224663406848));
#60511=CARTESIAN_POINT('Ctrl Pts',(12.2711805139213,-17.0828938614663,78.4968565980093));
#60512=CARTESIAN_POINT('Ctrl Pts',(12.2706690975431,-17.0850329711507,78.4999086084107));
#60513=CARTESIAN_POINT('Ctrl Pts',(12.2614414961737,-17.1228243859493,78.5544769284436));
#60514=CARTESIAN_POINT('Ctrl Pts',(12.228036692318,-17.218306148821,78.7260201971924));
#60515=CARTESIAN_POINT('Ctrl Pts',(12.1731938226851,-17.2549658653676,78.9122669584772));
#60516=CARTESIAN_POINT('Ctrl Pts',(12.0925286612292,-17.2551291983681,79.1341301729733));
#60517=CARTESIAN_POINT('Ctrl Pts',(12.0139885788277,-17.2197201593246,79.3155689316349));
#60518=CARTESIAN_POINT('Ctrl Pts',(11.929324830863,-17.1256354200658,79.4690811831062));
#60519=CARTESIAN_POINT('Ctrl Pts',(11.8979359134617,-17.0829544530057,79.5224663406848));
#60520=CARTESIAN_POINT('Ctrl Pts',(11.8979359134617,-17.0829544530057,79.5224663406848));
#60521=CARTESIAN_POINT('Ctrl Pts',(11.8797818085212,-17.0582694743852,79.5533421985731));
#60522=CARTESIAN_POINT('Ctrl Pts',(11.862111845529,-17.0315136611155,79.5821596885964));
#60523=CARTESIAN_POINT('Ctrl Pts',(11.8340060584782,-16.9839356481672,79.626485701499));
#60524=CARTESIAN_POINT('Ctrl Pts',(11.822863335852,-16.9636835154004,79.6436043679924));
#60525=CARTESIAN_POINT('Ctrl Pts',(11.7419583042977,-16.8055520460372,79.7657541392426));
#60526=CARTESIAN_POINT('Ctrl Pts',(11.6322385355776,-16.4531466810754,79.9023659741719));
#60527=CARTESIAN_POINT('Ctrl Pts',(11.6852150750259,-15.9157775367878,79.8401596355449));
#60528=CARTESIAN_POINT('Ctrl Pts',(11.8251071448527,-15.616984349081,79.6451820555524));
#60529=CARTESIAN_POINT('Ctrl Pts',(11.9811196883727,-15.4003238547929,79.3825863055803));
#60530=CARTESIAN_POINT('Ctrl Pts',(12.0821287866527,-15.3383729044183,79.1685196844361));
#60531=CARTESIAN_POINT('Ctrl Pts',(12.1440294707702,-15.3457361617732,78.9916063779574));
#60532=CARTESIAN_POINT('Origin',(14.2351639486941,-16.3,79.7926130762057));
#60533=CARTESIAN_POINT('',(16.4513530905785,-16.3,79.7425768505124));
#60534=CARTESIAN_POINT('Ctrl Pts',(16.4513530905785,-16.3,79.7425768505124));
#60535=CARTESIAN_POINT('Ctrl Pts',(16.4513530905785,-16.3589692886209,79.7425768505124));
#60536=CARTESIAN_POINT('Ctrl Pts',(16.4480480854555,-16.4816735726619,79.7558601913112));
#60537=CARTESIAN_POINT('Ctrl Pts',(16.4325736298389,-16.6594622572905,79.8171984098592));
#60538=CARTESIAN_POINT('Ctrl Pts',(16.4062748363779,-16.8159706118973,79.9166929639477));
#60539=CARTESIAN_POINT('Ctrl Pts',(16.3729890665525,-16.9364358562187,80.0357782635816));
#60540=CARTESIAN_POINT('Ctrl Pts',(16.3356911646629,-17.0179798530874,80.1605114661715));
#60541=CARTESIAN_POINT('Ctrl Pts',(16.3058473255403,-17.0575804523145,80.254295100986));
#60542=CARTESIAN_POINT('Ctrl Pts',(16.2879525013642,-17.0755371418863,80.308927696043));
#60543=CARTESIAN_POINT('Ctrl Pts',(16.2415372469172,-17.1117868061966,80.447753029014));
#60544=CARTESIAN_POINT('Ctrl Pts',(16.1948063223941,-17.1115730952314,80.576147720836));
#60545=CARTESIAN_POINT('Ctrl Pts',(16.1449618162535,-17.0790101292845,80.7029348679748));
#60546=CARTESIAN_POINT('Ctrl Pts',(16.1307085706017,-17.0681960618883,80.7387696350713));
#60547=CARTESIAN_POINT('Ctrl Pts',(16.1056532177054,-17.0453545991598,80.800704934583));
#60548=CARTESIAN_POINT('Ctrl Pts',(16.0703540029782,-17.0022330082117,80.8851607398882));
#60549=CARTESIAN_POINT('Ctrl Pts',(16.0301839042296,-16.9342077983924,80.9775549085599));
#60550=CARTESIAN_POINT('Ctrl Pts',(15.9832611827489,-16.8301442655337,81.0820269634397));
#60551=CARTESIAN_POINT('Ctrl Pts',(15.9502407645414,-16.7212601418262,81.1524384808638));
#60552=CARTESIAN_POINT('Ctrl Pts',(15.9312021587559,-16.6273889065201,81.1923360286486));
#60553=CARTESIAN_POINT('Ctrl Pts',(15.9241925939478,-16.5891969664984,81.2069681165303));
#60554=CARTESIAN_POINT('Ctrl Pts',(15.9165903821184,-16.5402506433046,81.2227467611148));
#60555=CARTESIAN_POINT('Ctrl Pts',(15.91065385941,-16.4902046723651,81.2349960729889));
#60556=CARTESIAN_POINT('Ctrl Pts',(15.9069299685908,-16.4499097222704,81.2426581791741));
#60557=CARTESIAN_POINT('Ctrl Pts',(15.8993860003837,-16.3486391820234,81.2581428999399));
#60558=CARTESIAN_POINT('Ctrl Pts',(15.8993339911057,-16.2514057238454,81.2582653088229));
#60559=CARTESIAN_POINT('Ctrl Pts',(15.9068883109817,-16.1499522168206,81.2427575723468));
#60560=CARTESIAN_POINT('Ctrl Pts',(15.9106060634705,-16.1096920097338,81.2351100583515));
#60561=CARTESIAN_POINT('Ctrl Pts',(15.9189462667354,-16.039575969747,81.2178946689264));
#60562=CARTESIAN_POINT('Ctrl Pts',(15.9390487495246,-15.9236171521494,81.176123768719));
#60563=CARTESIAN_POINT('Ctrl Pts',(15.9780188589416,-15.7841245162218,81.093298797813));
#60564=CARTESIAN_POINT('Ctrl Pts',(16.0206262002669,-15.6838578074055,80.9992772183258));
#60565=CARTESIAN_POINT('Ctrl Pts',(16.0601083842914,-15.614453165806,80.9088149092774));
#60566=CARTESIAN_POINT('Ctrl Pts',(16.0913245109124,-15.5711026393277,80.8352208082551));
#60567=CARTESIAN_POINT('Ctrl Pts',(16.1140619626514,-15.5467976611288,80.7799456784944));
#60568=CARTESIAN_POINT('Ctrl Pts',(16.1274512959284,-15.5348564441079,80.7467731693007));
#60569=CARTESIAN_POINT('Ctrl Pts',(16.1328072862571,-15.5302830340556,80.7334485354894));
#60570=CARTESIAN_POINT('Ctrl Pts',(16.1381613217313,-15.5260194401552,80.7200442157294));
#60571=CARTESIAN_POINT('Ctrl Pts',(16.1435063115107,-15.5220675070163,80.7065768755647));
#60572=CARTESIAN_POINT('Ctrl Pts',(16.1475083522864,-15.5192597790203,80.6964500598804));
#60573=CARTESIAN_POINT('Ctrl Pts',(16.1508391816247,-15.5170502299053,80.6879848666869));
#60574=CARTESIAN_POINT('Ctrl Pts',(16.15349609922,-15.5153610551317,80.6812109984591));
#60575=CARTESIAN_POINT('Ctrl Pts',(16.1761138473566,-15.5014438248939,80.6234102411006));
#60576=CARTESIAN_POINT('Ctrl Pts',(16.2173799719997,-15.4890669000081,80.5140466644355));
#60577=CARTESIAN_POINT('Ctrl Pts',(16.256671069509,-15.5016526498119,80.4020055506128));
#60578=CARTESIAN_POINT('Ctrl Pts',(16.2776453806387,-15.5166287131285,80.339710128914));
#60579=CARTESIAN_POINT('Ctrl Pts',(16.2822621877799,-15.5201625714385,80.3259280683213));
#60580=CARTESIAN_POINT('Ctrl Pts',(16.2902787106003,-15.5269026562889,80.3018213429743));
#60581=CARTESIAN_POINT('Ctrl Pts',(16.3059640273659,-15.5425274630872,80.253955052204));
#60582=CARTESIAN_POINT('Ctrl Pts',(16.3272838914141,-15.5711106544873,80.1869069342357));
#60583=CARTESIAN_POINT('Ctrl Pts',(16.3506559088329,-15.6144081339517,80.1105373437524));
#60584=CARTESIAN_POINT('Ctrl Pts',(16.3786675677716,-15.6840040800632,80.0154883579624));
#60585=CARTESIAN_POINT('Ctrl Pts',(16.3965034681242,-15.7486486439767,79.9516745085037));
#60586=CARTESIAN_POINT('Ctrl Pts',(16.4088407689086,-15.8075043665704,79.9062850349126));
#60587=CARTESIAN_POINT('Ctrl Pts',(16.413584292267,-15.8316774627009,79.8887037060206));
#60588=CARTESIAN_POINT('Ctrl Pts',(16.4214143032745,-15.8757440839149,79.8594045459933));
#60589=CARTESIAN_POINT('Ctrl Pts',(16.4428541971365,-16.0236308749458,79.7774158873755));
#60590=CARTESIAN_POINT('Ctrl Pts',(16.4513530905785,-16.1820614227582,79.7425768505124));
#60591=CARTESIAN_POINT('Ctrl Pts',(16.4513530905785,-16.3,79.7425768505124));
#60592=CARTESIAN_POINT('',(14.5104901640713,-16.3,79.036160516473));
#60593=CARTESIAN_POINT('Origin',(9.31,-16.425,78.));
#60594=CARTESIAN_POINT('',(6.3075,-18.7,78.));
#60595=CARTESIAN_POINT('Origin',(9.31,-18.7,78.));
#60596=CARTESIAN_POINT('',(6.3075,-14.15,78.));
#60597=CARTESIAN_POINT('',(6.3075,-16.425,78.));
#60598=CARTESIAN_POINT('Origin',(9.31,-14.15,78.));
#60599=CARTESIAN_POINT('Ctrl Pts',(16.6267263258151,-16.3,79.647882238852));
#60600=CARTESIAN_POINT('Ctrl Pts',(16.6267263258151,-16.3686398740138,79.647882238852));
#60601=CARTESIAN_POINT('Ctrl Pts',(16.6232895344097,-16.5114662207145,79.6631181782204));
#60602=CARTESIAN_POINT('Ctrl Pts',(16.6070569699324,-16.7195440420054,79.7337450825527));
#60603=CARTESIAN_POINT('Ctrl Pts',(16.5787193153288,-16.9047265894586,79.8495489824192));
#60604=CARTESIAN_POINT('Ctrl Pts',(16.5417979890631,-17.0491114348861,79.9898247024023));
#60605=CARTESIAN_POINT('Ctrl Pts',(16.4991469954625,-17.1481299251104,80.1385791791468));
#60606=CARTESIAN_POINT('Ctrl Pts',(16.4642217393025,-17.1966318363056,80.251361487145));
#60607=CARTESIAN_POINT('Ctrl Pts',(16.4430881666924,-17.2186801784522,80.3172431103551));
#60608=CARTESIAN_POINT('Ctrl Pts',(16.3879482597749,-17.2633110844262,80.4849293868592));
#60609=CARTESIAN_POINT('Ctrl Pts',(16.3311939963963,-17.263076777122,80.640871035239));
#60610=CARTESIAN_POINT('Ctrl Pts',(16.2703393347549,-17.2229799642533,80.7935103025339));
#60611=CARTESIAN_POINT('Ctrl Pts',(16.2529286652786,-17.2096866928451,80.8365863008715));
#60612=CARTESIAN_POINT('Ctrl Pts',(16.2223085872669,-17.1816622921672,80.9108472236554));
#60613=CARTESIAN_POINT('Ctrl Pts',(16.1791754703243,-17.1289822618776,81.0115059847778));
#60614=CARTESIAN_POINT('Ctrl Pts',(16.1302272700693,-17.0466007917327,81.1205411519808));
#60615=CARTESIAN_POINT('Ctrl Pts',(16.0732729417727,-16.9216470840919,81.2426097135714));
#60616=CARTESIAN_POINT('Ctrl Pts',(16.0334936810962,-16.7925239444982,81.3235736952026));
#60617=CARTESIAN_POINT('Ctrl Pts',(16.0106538593799,-16.6821981103206,81.3691011936988));
#60618=CARTESIAN_POINT('Ctrl Pts',(16.0022521358187,-16.6373793785181,81.3857696123251));
#60619=CARTESIAN_POINT('Ctrl Pts',(15.9931529411453,-16.5800659147356,81.4036970257625));
#60620=CARTESIAN_POINT('Ctrl Pts',(15.9860578245946,-16.5216040414588,81.4175766075504));
#60621=CARTESIAN_POINT('Ctrl Pts',(15.9816103595508,-16.4745965934211,81.4262469365913));
#60622=CARTESIAN_POINT('Ctrl Pts',(15.9726062552113,-16.3565449674897,81.443748920257));
#60623=CARTESIAN_POINT('Ctrl Pts',(15.9725425009045,-16.2435059768007,81.4438943965471));
#60624=CARTESIAN_POINT('Ctrl Pts',(15.981559283011,-16.1252411321897,81.4263653146201));
#60625=CARTESIAN_POINT('Ctrl Pts',(15.9859992260481,-16.0782746472634,81.4177123723923));
#60626=CARTESIAN_POINT('Ctrl Pts',(15.9959680144551,-15.996365623908,81.3982024054527));
#60627=CARTESIAN_POINT('Ctrl Pts',(16.0200372266792,-15.8604273231654,81.3507157648354));
#60628=CARTESIAN_POINT('Ctrl Pts',(16.0669428124562,-15.6953850753735,81.2556190750553));
#60629=CARTESIAN_POINT('Ctrl Pts',(16.1185975434662,-15.5751968380705,81.1460824099368));
#60630=CARTESIAN_POINT('Ctrl Pts',(16.1666865284266,-15.4912543308356,81.0394472234925));
#60631=CARTESIAN_POINT('Ctrl Pts',(16.2047961808524,-15.4384721428059,80.952041722185));
#60632=CARTESIAN_POINT('Ctrl Pts',(16.2325860018634,-15.4087182634758,80.8859576775251));
#60633=CARTESIAN_POINT('Ctrl Pts',(16.248947338163,-15.3940656126707,80.8461713540943));
#60634=CARTESIAN_POINT('Ctrl Pts',(16.2554916800538,-15.388450767397,80.8301796061662));
#60635=CARTESIAN_POINT('Ctrl Pts',(16.2620326141532,-15.3832121080572,80.8140766685934));
#60636=CARTESIAN_POINT('Ctrl Pts',(16.2685609643578,-15.3783529418162,80.7978834589029));
#60637=CARTESIAN_POINT('Ctrl Pts',(16.2734481412606,-15.3748990742495,80.7856999038481));
#60638=CARTESIAN_POINT('Ctrl Pts',(16.2775147617408,-15.3721798545712,80.7755097810832));
#60639=CARTESIAN_POINT('Ctrl Pts',(16.2807580438145,-15.37010041347,80.7673524199429));
#60640=CARTESIAN_POINT('Ctrl Pts',(16.308363242307,-15.3529640814669,80.6977276874573));
#60641=CARTESIAN_POINT('Ctrl Pts',(16.3586107169648,-15.3376504708956,80.5654454852136));
#60642=CARTESIAN_POINT('Ctrl Pts',(16.4058754210574,-15.353224391122,80.4297068102671));
#60643=CARTESIAN_POINT('Ctrl Pts',(16.4308398851589,-15.371663215768,80.3544280421398));
#60644=CARTESIAN_POINT('Ctrl Pts',(16.4363274974597,-15.3760122112162,80.3377790265208));
#60645=CARTESIAN_POINT('Ctrl Pts',(16.4458365951828,-15.3843016285567,80.3086730273532));
#60646=CARTESIAN_POINT('Ctrl Pts',(16.4643631140139,-15.4034928690422,80.2509476732841));
#60647=CARTESIAN_POINT('Ctrl Pts',(16.4893053796703,-15.438486627179,80.1703295926858));
#60648=CARTESIAN_POINT('Ctrl Pts',(16.5162719674538,-15.4912042488478,80.0789622080761));
#60649=CARTESIAN_POINT('Ctrl Pts',(16.548100587601,-15.5753837738119,79.9659216531079));
#60650=CARTESIAN_POINT('Ctrl Pts',(16.5678845354643,-15.6528601133616,79.8907518590427));
#60651=CARTESIAN_POINT('Ctrl Pts',(16.5813766158318,-15.7228477592171,79.837607390227));
#60652=CARTESIAN_POINT('Ctrl Pts',(16.586544255709,-15.7515481629588,79.8170540818662));
#60653=CARTESIAN_POINT('Ctrl Pts',(16.5950312459286,-15.8037451346603,79.7828728219127));
#60654=CARTESIAN_POINT('Ctrl Pts',(16.6179955133542,-15.9782014756465,79.6876782461328));
#60655=CARTESIAN_POINT('Ctrl Pts',(16.6267263258151,-16.1627202519724,79.6478822388519));
#60656=CARTESIAN_POINT('Ctrl Pts',(16.6267263258151,-16.3,79.6478822388519));
#60657=CARTESIAN_POINT('Ctrl Pts',(16.5682685807363,-16.3,79.6794471094054));
#60658=CARTESIAN_POINT('Ctrl Pts',(16.5682685807363,-16.3654163455495,79.6794471094054));
#60659=CARTESIAN_POINT('Ctrl Pts',(16.5648757180916,-16.5015353380303,79.694032182584));
#60660=CARTESIAN_POINT('Ctrl Pts',(16.5488958565679,-16.6995167804338,79.7615628583216));
#60661=CARTESIAN_POINT('Ctrl Pts',(16.5212378223452,-16.8751412636049,79.8719303095954));
#60662=CARTESIAN_POINT('Ctrl Pts',(16.4855283482262,-17.0115529086637,80.0051425561287));
#60663=CARTESIAN_POINT('Ctrl Pts',(16.4446617185293,-17.1047465677694,80.1458899414884));
#60664=CARTESIAN_POINT('Ctrl Pts',(16.4114302680484,-17.1502813749753,80.2523393584253));
#60665=CARTESIAN_POINT('Ctrl Pts',(16.3913762782497,-17.1709658329303,80.3144713055844));
#60666=CARTESIAN_POINT('Ctrl Pts',(16.3391445888223,-17.212802991683,80.4725372675774));
#60667=CARTESIAN_POINT('Ctrl Pts',(16.2857314383956,-17.2125755498251,80.6192965971047));
#60668=CARTESIAN_POINT('Ctrl Pts',(16.2285468285878,-17.1749900192637,80.7633184910142));
#60669=CARTESIAN_POINT('Ctrl Pts',(16.2121886337196,-17.1625231491928,80.8039807456047));
#60670=CARTESIAN_POINT('Ctrl Pts',(16.1834234640797,-17.136226394498,80.8741331272979));
#60671=CARTESIAN_POINT('Ctrl Pts',(16.1429016478756,-17.0867325106556,80.9693909031479));
#60672=CARTESIAN_POINT('Ctrl Pts',(16.0968794814561,-17.0091364606193,81.0728790708405));
#60673=CARTESIAN_POINT('Ctrl Pts',(16.0432690220981,-16.8911461445725,81.1890821301941));
#60674=CARTESIAN_POINT('Ctrl Pts',(16.0057427089113,-16.7687693436075,81.2665286237563));
#60675=CARTESIAN_POINT('Ctrl Pts',(15.9841699591719,-16.6639283757204,81.3101794720153));
#60676=CARTESIAN_POINT('Ctrl Pts',(15.9762322885284,-16.6213185745115,81.3261691137268));
#60677=CARTESIAN_POINT('Ctrl Pts',(15.9676320881363,-16.5667941575919,81.3433802708799));
#60678=CARTESIAN_POINT('Ctrl Pts',(15.9609231695331,-16.5111375850943,81.3567164293632));
#60679=CARTESIAN_POINT('Ctrl Pts',(15.9567168958975,-16.4663676363709,81.3650506841189));
#60680=CARTESIAN_POINT('Ctrl Pts',(15.9481995036021,-16.3539097056676,81.3818802468179));
#60681=CARTESIAN_POINT('Ctrl Pts',(15.9481396643049,-16.2461392258156,81.3820180339724));
#60682=CARTESIAN_POINT('Ctrl Pts',(15.9566689590012,-16.1334781604,81.3651627338623));
#60683=CARTESIAN_POINT('Ctrl Pts',(15.9608681718556,-16.0887471014202,81.3568449343787));
#60684=CARTESIAN_POINT('Ctrl Pts',(15.9702940985485,-16.010769072521,81.3380998266106));
#60685=CARTESIAN_POINT('Ctrl Pts',(15.9930410676277,-15.8814905994934,81.2925184327966));
#60686=CARTESIAN_POINT('Ctrl Pts',(16.037301494618,-15.7249648889896,81.2015123159746));
#60687=CARTESIAN_POINT('Ctrl Pts',(16.0859404290664,-15.6114171611822,81.0971473460665));
#60688=CARTESIAN_POINT('Ctrl Pts',(16.1311604803816,-15.5323206091591,80.9959031187542));
#60689=CARTESIAN_POINT('Ctrl Pts',(16.1669722908724,-15.4826823083131,80.9131014175417));
#60690=CARTESIAN_POINT('Ctrl Pts',(16.1930779887927,-15.4547447293601,80.8506203445149));
#60691=CARTESIAN_POINT('Ctrl Pts',(16.2084486574181,-15.4409958898165,80.8130386258298));
#60692=CARTESIAN_POINT('Ctrl Pts',(16.2145968821216,-15.4357281896166,80.7979359159407));
#60693=CARTESIAN_POINT('Ctrl Pts',(16.2207421833459,-15.4308145520899,80.7827325176388));
#60694=CARTESIAN_POINT('Ctrl Pts',(16.2268760800755,-15.4262577968829,80.7674479311235));
#60695=CARTESIAN_POINT('Ctrl Pts',(16.2314682116025,-15.4230193091731,80.7559499558589));
#60696=CARTESIAN_POINT('Ctrl Pts',(16.2352895683688,-15.4204699796826,80.7463348096178));
#60697=CARTESIAN_POINT('Ctrl Pts',(16.2383373956163,-15.4185206273572,80.7386386127816));
#60698=CARTESIAN_POINT('Ctrl Pts',(16.2642801106568,-15.4024573292759,80.6729552053384));
#60699=CARTESIAN_POINT('Ctrl Pts',(16.3115338019764,-15.3881226139331,80.5483125449542));
#60700=CARTESIAN_POINT('Ctrl Pts',(16.3561406372079,-15.402700477352,80.420473057049));
#60701=CARTESIAN_POINT('Ctrl Pts',(16.3797750503189,-15.4199850482215,80.3495220710645));
#60702=CARTESIAN_POINT('Ctrl Pts',(16.3849723942331,-15.4240623312903,80.333828707121));
#60703=CARTESIAN_POINT('Ctrl Pts',(16.3939839669887,-15.4318353044674,80.3063891325602));
#60704=CARTESIAN_POINT('Ctrl Pts',(16.4115634184646,-15.4498377337239,80.2519501329241));
#60705=CARTESIAN_POINT('Ctrl Pts',(16.4352982169183,-15.4826946362818,80.1758553732025));
#60706=CARTESIAN_POINT('Ctrl Pts',(16.4610666145802,-15.5322722105491,80.0894872533015));
#60707=CARTESIAN_POINT('Ctrl Pts',(16.4916229143245,-15.6115905425624,79.9824438880594));
#60708=CARTESIAN_POINT('Ctrl Pts',(16.5107575130176,-15.6847896235666,79.911059408863));
#60709=CARTESIAN_POINT('Ctrl Pts',(16.5238646668574,-15.7510666283349,79.8604999384555));
#60710=CARTESIAN_POINT('Ctrl Pts',(16.5288909345617,-15.7782579295395,79.8409372899176));
#60711=CARTESIAN_POINT('Ctrl Pts',(16.5371589317105,-15.8277447844118,79.8083833966062));
#60712=CARTESIAN_POINT('Ctrl Pts',(16.559615074615,-15.9933446087463,79.7175907932137));
#60713=CARTESIAN_POINT('Ctrl Pts',(16.5682685807363,-16.169167308901,79.6794471094054));
#60714=CARTESIAN_POINT('Ctrl Pts',(16.5682685807363,-16.3,79.6794471094054));
#60715=CARTESIAN_POINT('Ctrl Pts',(16.5098108356574,-16.3,79.7110119799589));
#60716=CARTESIAN_POINT('Ctrl Pts',(16.5098108356574,-16.3621928170852,79.7110119799589));
#60717=CARTESIAN_POINT('Ctrl Pts',(16.5064619017735,-16.4916044553461,79.7249461869476));
#60718=CARTESIAN_POINT('Ctrl Pts',(16.4907347432034,-16.6794895188621,79.7893806340904));
#60719=CARTESIAN_POINT('Ctrl Pts',(16.4637563293615,-16.8455559377511,79.8943116367715));
#60720=CARTESIAN_POINT('Ctrl Pts',(16.4292587073893,-16.9739943824412,80.0204604098552));
#60721=CARTESIAN_POINT('Ctrl Pts',(16.3901764415961,-17.0613632104284,80.15320070383));
#60722=CARTESIAN_POINT('Ctrl Pts',(16.3586387967944,-17.1039309136449,80.2533172297057));
#60723=CARTESIAN_POINT('Ctrl Pts',(16.3396643898069,-17.1232514874083,80.3116995008137));
#60724=CARTESIAN_POINT('Ctrl Pts',(16.2903409178698,-17.1622948989398,80.4601451482957));
#60725=CARTESIAN_POINT('Ctrl Pts',(16.2402688803948,-17.1620743225282,80.5977221589703));
#60726=CARTESIAN_POINT('Ctrl Pts',(16.1867543224206,-17.1270000742741,80.7331266794945));
#60727=CARTESIAN_POINT('Ctrl Pts',(16.1714486021607,-17.1153596055406,80.771375190338));
#60728=CARTESIAN_POINT('Ctrl Pts',(16.1445383408925,-17.0907904968289,80.8374190309404));
#60729=CARTESIAN_POINT('Ctrl Pts',(16.1066278254269,-17.0444827594336,80.9272758215181));
#60730=CARTESIAN_POINT('Ctrl Pts',(16.0635316928428,-16.9716721295058,81.0252169897002));
#60731=CARTESIAN_POINT('Ctrl Pts',(16.0132651024235,-16.8606452050531,81.1355545468169));
#60732=CARTESIAN_POINT('Ctrl Pts',(15.9779917367264,-16.7450147427169,81.20948355231));
#60733=CARTESIAN_POINT('Ctrl Pts',(15.9576860589639,-16.6456586411203,81.2512577503319));
#60734=CARTESIAN_POINT('Ctrl Pts',(15.9502124412381,-16.605257770505,81.2665686151285));
#60735=CARTESIAN_POINT('Ctrl Pts',(15.9421112351274,-16.5535224004483,81.2830635159973));
#60736=CARTESIAN_POINT('Ctrl Pts',(15.9357885144715,-16.5006711287297,81.295856251176));
#60737=CARTESIAN_POINT('Ctrl Pts',(15.9318234322441,-16.4581386793206,81.3038544316465));
#60738=CARTESIAN_POINT('Ctrl Pts',(15.9237927519929,-16.3512744438455,81.3200115733789));
#60739=CARTESIAN_POINT('Ctrl Pts',(15.9237368277053,-16.2487724748305,81.3201416713976));
#60740=CARTESIAN_POINT('Ctrl Pts',(15.9317786349915,-16.1417151886103,81.3039601531045));
#60741=CARTESIAN_POINT('Ctrl Pts',(15.935737117663,-16.099219555577,81.2959774963651));
#60742=CARTESIAN_POINT('Ctrl Pts',(15.9446201826419,-16.025172521134,81.2779972477685));
#60743=CARTESIAN_POINT('Ctrl Pts',(15.9660449085761,-15.9025538758214,81.2343211007578));
#60744=CARTESIAN_POINT('Ctrl Pts',(16.0076601767798,-15.7545447026057,81.1474055568938));
#60745=CARTESIAN_POINT('Ctrl Pts',(16.0532833146667,-15.6476374842939,81.0482122821961));
#60746=CARTESIAN_POINT('Ctrl Pts',(16.0956344323365,-15.5733868874825,80.9523590140158));
#60747=CARTESIAN_POINT('Ctrl Pts',(16.1291484008924,-15.5268924738204,80.8741611128984));
#60748=CARTESIAN_POINT('Ctrl Pts',(16.153569975722,-15.5007711952445,80.8152830115046));
#60749=CARTESIAN_POINT('Ctrl Pts',(16.1679499766733,-15.4879261669622,80.7799058975652));
#60750=CARTESIAN_POINT('Ctrl Pts',(16.1737020841893,-15.4830056118361,80.765692225715));
#60751=CARTESIAN_POINT('Ctrl Pts',(16.1794517525386,-15.4784169961225,80.7513883666841));
#60752=CARTESIAN_POINT('Ctrl Pts',(16.1851911957931,-15.4741626519496,80.7370124033441));
#60753=CARTESIAN_POINT('Ctrl Pts',(16.1894882819445,-15.4711395440967,80.7262000078696));
#60754=CARTESIAN_POINT('Ctrl Pts',(16.1930643749967,-15.468760104794,80.7171598381523));
#60755=CARTESIAN_POINT('Ctrl Pts',(16.1959167474182,-15.4669408412445,80.7099248056204));
#60756=CARTESIAN_POINT('Ctrl Pts',(16.2201969790067,-15.4519505770849,80.6481827232194));
#60757=CARTESIAN_POINT('Ctrl Pts',(16.2644568869881,-15.4385947569706,80.5311796046948));
#60758=CARTESIAN_POINT('Ctrl Pts',(16.3064058533584,-15.4521765635819,80.411239303831));
#60759=CARTESIAN_POINT('Ctrl Pts',(16.3287102154788,-15.468306880675,80.3446160999893));
#60760=CARTESIAN_POINT('Ctrl Pts',(16.3336172910065,-15.4721124513644,80.3298783877211));
#60761=CARTESIAN_POINT('Ctrl Pts',(16.3421313387945,-15.4793689803781,80.3041052377673));
#60762=CARTESIAN_POINT('Ctrl Pts',(16.3587637229153,-15.4961825984056,80.2529525925641));
#60763=CARTESIAN_POINT('Ctrl Pts',(16.3812910541662,-15.5269026453845,80.1813811537191));
#60764=CARTESIAN_POINT('Ctrl Pts',(16.4058612617066,-15.5733401722504,80.100012298527));
#60765=CARTESIAN_POINT('Ctrl Pts',(16.4351452410481,-15.6477973113128,79.9989661230109));
#60766=CARTESIAN_POINT('Ctrl Pts',(16.4536304905709,-15.7167191337717,79.9313669586834));
#60767=CARTESIAN_POINT('Ctrl Pts',(16.466352717883,-15.7792854974526,79.8833924866841));
#60768=CARTESIAN_POINT('Ctrl Pts',(16.4712376134143,-15.8049676961202,79.8648204979691));
#60769=CARTESIAN_POINT('Ctrl Pts',(16.4792866174925,-15.8517444341634,79.8338939712997));
#60770=CARTESIAN_POINT('Ctrl Pts',(16.5012346358758,-16.0084877418461,79.7475033402946));
#60771=CARTESIAN_POINT('Ctrl Pts',(16.5098108356574,-16.1756143658296,79.7110119799589));
#60772=CARTESIAN_POINT('Ctrl Pts',(16.5098108356574,-16.3,79.7110119799589));
#60773=CARTESIAN_POINT('Ctrl Pts',(16.4513530905785,-16.3,79.7425768505124));
#60774=CARTESIAN_POINT('Ctrl Pts',(16.4513530905785,-16.3589692886209,79.7425768505124));
#60775=CARTESIAN_POINT('Ctrl Pts',(16.4480480854555,-16.4816735726619,79.7558601913112));
#60776=CARTESIAN_POINT('Ctrl Pts',(16.4325736298389,-16.6594622572905,79.8171984098592));
#60777=CARTESIAN_POINT('Ctrl Pts',(16.4062748363779,-16.8159706118973,79.9166929639477));
#60778=CARTESIAN_POINT('Ctrl Pts',(16.3729890665525,-16.9364358562187,80.0357782635816));
#60779=CARTESIAN_POINT('Ctrl Pts',(16.3356911646629,-17.0179798530874,80.1605114661715));
#60780=CARTESIAN_POINT('Ctrl Pts',(16.3058473255403,-17.0575804523145,80.254295100986));
#60781=CARTESIAN_POINT('Ctrl Pts',(16.2879525013642,-17.0755371418863,80.308927696043));
#60782=CARTESIAN_POINT('Ctrl Pts',(16.2415372469172,-17.1117868061966,80.447753029014));
#60783=CARTESIAN_POINT('Ctrl Pts',(16.1948063223941,-17.1115730952314,80.576147720836));
#60784=CARTESIAN_POINT('Ctrl Pts',(16.1449618162535,-17.0790101292845,80.7029348679748));
#60785=CARTESIAN_POINT('Ctrl Pts',(16.1307085706017,-17.0681960618883,80.7387696350713));
#60786=CARTESIAN_POINT('Ctrl Pts',(16.1056532177054,-17.0453545991598,80.800704934583));
#60787=CARTESIAN_POINT('Ctrl Pts',(16.0703540029782,-17.0022330082117,80.8851607398882));
#60788=CARTESIAN_POINT('Ctrl Pts',(16.0301839042296,-16.9342077983924,80.9775549085599));
#60789=CARTESIAN_POINT('Ctrl Pts',(15.9832611827489,-16.8301442655337,81.0820269634397));
#60790=CARTESIAN_POINT('Ctrl Pts',(15.9502407645414,-16.7212601418262,81.1524384808638));
#60791=CARTESIAN_POINT('Ctrl Pts',(15.9312021587559,-16.6273889065201,81.1923360286486));
#60792=CARTESIAN_POINT('Ctrl Pts',(15.9241925939478,-16.5891969664984,81.2069681165303));
#60793=CARTESIAN_POINT('Ctrl Pts',(15.9165903821184,-16.5402506433046,81.2227467611148));
#60794=CARTESIAN_POINT('Ctrl Pts',(15.91065385941,-16.4902046723651,81.2349960729889));
#60795=CARTESIAN_POINT('Ctrl Pts',(15.9069299685908,-16.4499097222704,81.2426581791741));
#60796=CARTESIAN_POINT('Ctrl Pts',(15.8993860003837,-16.3486391820234,81.2581428999399));
#60797=CARTESIAN_POINT('Ctrl Pts',(15.8993339911057,-16.2514057238454,81.2582653088229));
#60798=CARTESIAN_POINT('Ctrl Pts',(15.9068883109817,-16.1499522168206,81.2427575723468));
#60799=CARTESIAN_POINT('Ctrl Pts',(15.9106060634705,-16.1096920097338,81.2351100583515));
#60800=CARTESIAN_POINT('Ctrl Pts',(15.9189462667354,-16.039575969747,81.2178946689264));
#60801=CARTESIAN_POINT('Ctrl Pts',(15.9390487495246,-15.9236171521494,81.176123768719));
#60802=CARTESIAN_POINT('Ctrl Pts',(15.9780188589416,-15.7841245162218,81.093298797813));
#60803=CARTESIAN_POINT('Ctrl Pts',(16.0206262002669,-15.6838578074055,80.9992772183258));
#60804=CARTESIAN_POINT('Ctrl Pts',(16.0601083842914,-15.614453165806,80.9088149092774));
#60805=CARTESIAN_POINT('Ctrl Pts',(16.0913245109124,-15.5711026393277,80.8352208082551));
#60806=CARTESIAN_POINT('Ctrl Pts',(16.1140619626514,-15.5467976611288,80.7799456784944));
#60807=CARTESIAN_POINT('Ctrl Pts',(16.1274512959284,-15.5348564441079,80.7467731693007));
#60808=CARTESIAN_POINT('Ctrl Pts',(16.1328072862571,-15.5302830340556,80.7334485354894));
#60809=CARTESIAN_POINT('Ctrl Pts',(16.1381613217313,-15.5260194401552,80.7200442157294));
#60810=CARTESIAN_POINT('Ctrl Pts',(16.1435063115107,-15.5220675070163,80.7065768755647));
#60811=CARTESIAN_POINT('Ctrl Pts',(16.1475083522864,-15.5192597790203,80.6964500598804));
#60812=CARTESIAN_POINT('Ctrl Pts',(16.1508391816247,-15.5170502299053,80.6879848666869));
#60813=CARTESIAN_POINT('Ctrl Pts',(16.15349609922,-15.5153610551317,80.6812109984591));
#60814=CARTESIAN_POINT('Ctrl Pts',(16.1761138473566,-15.5014438248939,80.6234102411006));
#60815=CARTESIAN_POINT('Ctrl Pts',(16.2173799719997,-15.4890669000081,80.5140466644355));
#60816=CARTESIAN_POINT('Ctrl Pts',(16.256671069509,-15.5016526498119,80.4020055506128));
#60817=CARTESIAN_POINT('Ctrl Pts',(16.2776453806387,-15.5166287131285,80.339710128914));
#60818=CARTESIAN_POINT('Ctrl Pts',(16.2822621877799,-15.5201625714385,80.3259280683213));
#60819=CARTESIAN_POINT('Ctrl Pts',(16.2902787106003,-15.5269026562889,80.3018213429743));
#60820=CARTESIAN_POINT('Ctrl Pts',(16.3059640273659,-15.5425274630872,80.253955052204));
#60821=CARTESIAN_POINT('Ctrl Pts',(16.3272838914141,-15.5711106544873,80.1869069342357));
#60822=CARTESIAN_POINT('Ctrl Pts',(16.3506559088329,-15.6144081339517,80.1105373437524));
#60823=CARTESIAN_POINT('Ctrl Pts',(16.3786675677716,-15.6840040800632,80.0154883579624));
#60824=CARTESIAN_POINT('Ctrl Pts',(16.3965034681242,-15.7486486439767,79.9516745085037));
#60825=CARTESIAN_POINT('Ctrl Pts',(16.4088407689086,-15.8075043665704,79.9062850349126));
#60826=CARTESIAN_POINT('Ctrl Pts',(16.413584292267,-15.8316774627009,79.8887037060206));
#60827=CARTESIAN_POINT('Ctrl Pts',(16.4214143032745,-15.8757440839149,79.8594045459933));
#60828=CARTESIAN_POINT('Ctrl Pts',(16.4428541971365,-16.0236308749458,79.7774158873755));
#60829=CARTESIAN_POINT('Ctrl Pts',(16.4513530905785,-16.1820614227582,79.7425768505124));
#60830=CARTESIAN_POINT('Ctrl Pts',(16.4513530905785,-16.3,79.7425768505124));
#60831=CARTESIAN_POINT('',(16.6267263258151,-16.3,79.647882238852));
#60832=CARTESIAN_POINT('Origin',(10.315,-23.44,78.));
#60833=CARTESIAN_POINT('Origin',(10.315,-23.44,78.));
#60834=CARTESIAN_POINT('Origin',(12.3125,-18.7,78.));
#60835=CARTESIAN_POINT('Origin',(9.31,-14.1,78.));
#60836=CARTESIAN_POINT('',(6.2075,-14.05,78.));
#60837=CARTESIAN_POINT('',(6.2575,-14.1,78.));
#60838=CARTESIAN_POINT('Origin',(9.31,-14.05,78.));
#60839=CARTESIAN_POINT('Origin',(16.61,-14.05,78.));
#60840=CARTESIAN_POINT('',(2.01,-14.05,78.));
#60841=CARTESIAN_POINT('Origin',(9.31,-14.05,78.));
#60842=CARTESIAN_POINT('Origin',(9.31,-14.15,78.));
#60843=CARTESIAN_POINT('',(1.91,-14.15,78.));
#60844=CARTESIAN_POINT('Origin',(9.31,-25.4,78.));
#60845=CARTESIAN_POINT('',(1.91,-25.4,78.));
#70735=UNCERTAINTY_MEASURE_WITH_UNIT(LENGTH_MEASURE(0.001),#70758,
'DISTANCE_ACCURACY_VALUE',
'Maximum model space distance between geometric entities at asserted c
onnectivities');
#70740=UNCERTAINTY_MEASURE_WITH_UNIT(LENGTH_MEASURE(0.001),#70758,
'DISTANCE_ACCURACY_VALUE',
'Maximum model space distance between geometric entities at asserted c
onnectivities');
#70752=(
GEOMETRIC_REPRESENTATION_CONTEXT(3)
GLOBAL_UNCERTAINTY_ASSIGNED_CONTEXT((#70735))
GLOBAL_UNIT_ASSIGNED_CONTEXT((#70758,#70760,#70761))
REPRESENTATION_CONTEXT('','3D')
);
#70757=(
GEOMETRIC_REPRESENTATION_CONTEXT(3)
GLOBAL_UNCERTAINTY_ASSIGNED_CONTEXT((#70740))
GLOBAL_UNIT_ASSIGNED_CONTEXT((#70758,#70760,#70761))
REPRESENTATION_CONTEXT('','3D')
);
#70758=(
LENGTH_UNIT()
NAMED_UNIT(*)
SI_UNIT(.CENTI.,.METRE.)
);
#70760=(
NAMED_UNIT(*)
PLANE_ANGLE_UNIT()
SI_UNIT($,.RADIAN.)
);
#70761=(
NAMED_UNIT(*)
SI_UNIT($,.STERADIAN.)
SOLID_ANGLE_UNIT()
);
#70773=SHAPE_DEFINITION_REPRESENTATION(#70789,#70828);
#70789=PRODUCT_DEFINITION_SHAPE('',$,#70845);
#70828=SHAPE_REPRESENTATION('',(#27791),#70752);
#70833=PRODUCT_DEFINITION_CONTEXT('part definition',#70883,'design');
#70845=PRODUCT_DEFINITION('2026-10-19-02-58-13-081','04_D150_Lever_Hub',
#70861,#70833);
#70861=PRODUCT_DEFINITION_FORMATION('',$,#70896);
#70883=APPLICATION_CONTEXT(
'Core Data for Automotive Mechanical Design Process');
#70884=PRODUCT_CONTEXT('part definition',#70883,'mechanical');
#70896=PRODUCT('2026-10-19-02-58-13-081','04_D150_Lever_Hub',$,(#70884));
#71027=COLOUR_RGB('Light Blue',0.38,0.62,0.78);
#71028=FILL_AREA_STYLE_COLOUR('',#71027);
#71029=FILL_AREA_STYLE('',(#71028));
#71030=SURFACE_STYLE_FILL_AREA(#71029);
#71031=SURFACE_SIDE_STYLE('',(#71030));
#71032=SURFACE_STYLE_USAGE(.BOTH.,#71031);
#71033=PRESENTATION_STYLE_ASSIGNMENT((#71032));
ENDSEC;
END-ISO-10303-21;
